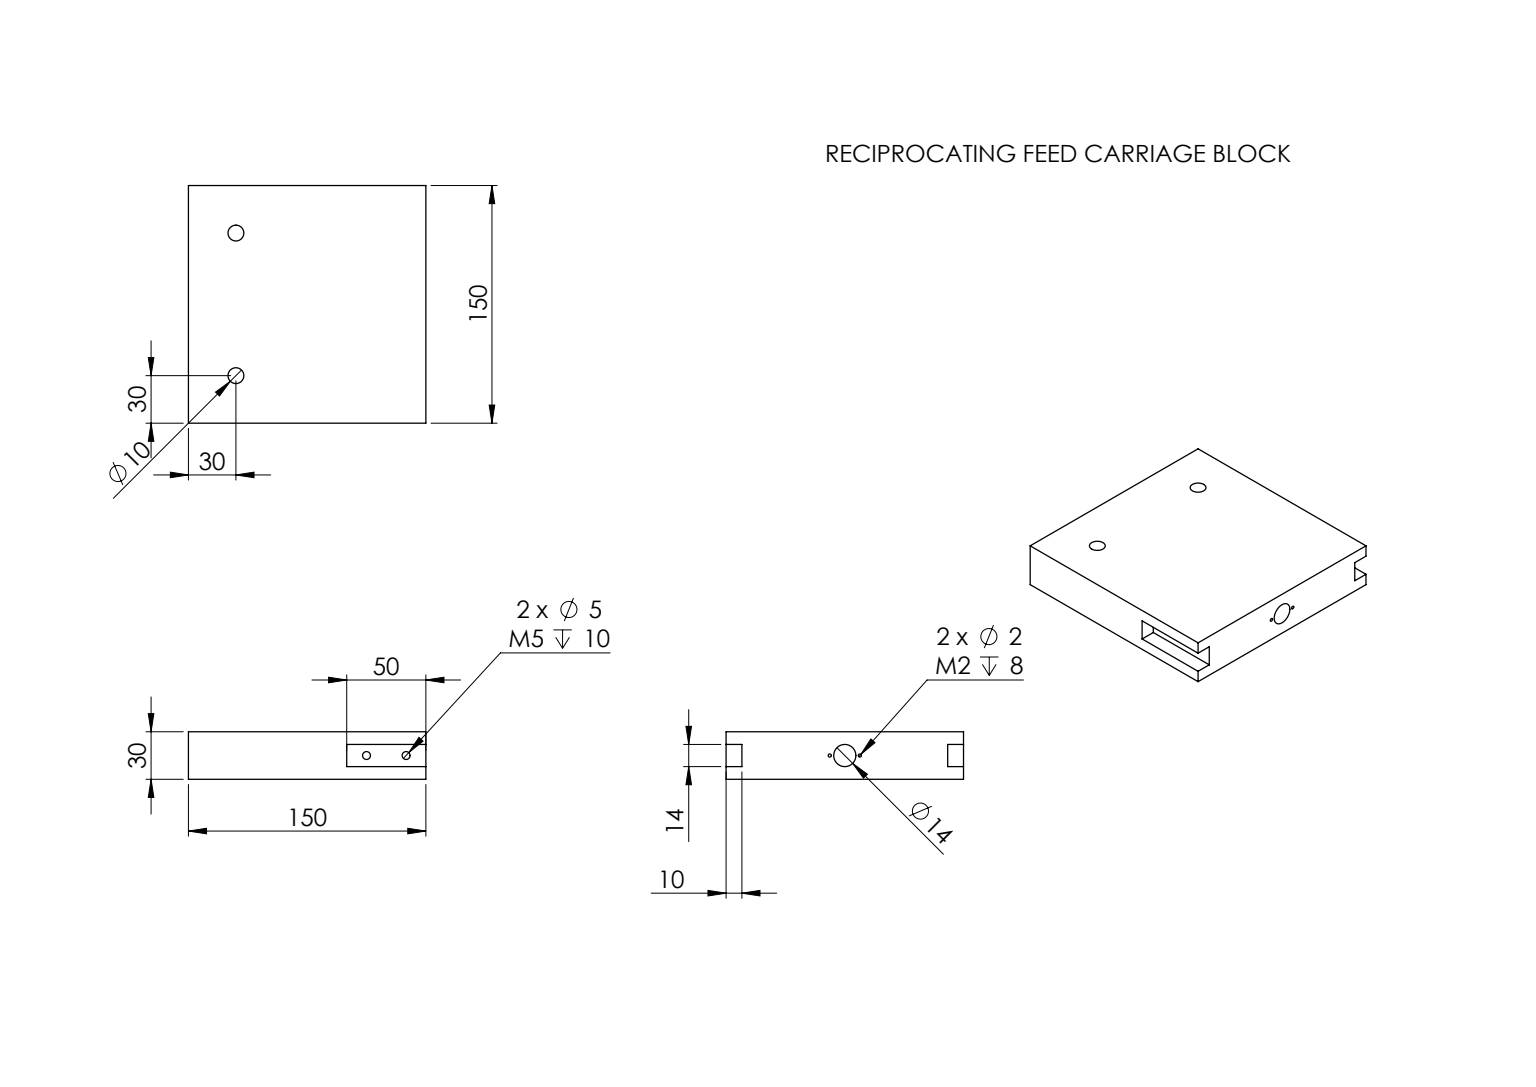
ISO-10303-21;
HEADER;
FILE_DESCRIPTION (('STEP AP214'),
    '1' );
FILE_NAME ('Reciprocating Feed Carriage Block.step',
    '2026-10-27T14:18:53',
    ( '' ),
    ( '' ),
    'SwSTEP 2.0',
    'SolidWorks 2026',
    '' );
FILE_SCHEMA (( 'AUTOMOTIVE_DESIGN' ));
ENDSEC;

DATA;
#3=LINE ( 'NONE', #3246, #2138 ) ;
#4=EDGE_LOOP ( 'NONE', ( #1502, #1673, #5385 ) ) ;
#6=FACE_BOUND ( 'NONE', #2071, .T. ) ;
#7=AXIS2_PLACEMENT_3D ( 'NONE', #5540, #5177, #924 ) ;
#19=DIRECTION ( 'NONE',  ( 0.8571673013836870192, 1.049727191973306873E-16, -0.5150380737757234151 ) ) ;
#21=VECTOR ( 'NONE', #291, 1000.000000000000000 ) ;
#22=EDGE_LOOP ( 'NONE', ( #259, #3713, #2794, #1342 ) ) ;
#23=ADVANCED_FACE ( 'NONE', ( #3966 ), #1603, .F. ) ;
#24=ORIENTED_EDGE ( 'NONE', *, *, #4586, .F. ) ;
#25=CIRCLE ( 'NONE', #2627, 2.500000000000002220 ) ;
#28=DIRECTION ( 'NONE',  ( 1.000000000000000000, -0.000000000000000000, -0.000000000000000000 ) ) ;
#30=CARTESIAN_POINT ( 'NONE',  ( 25.00000000000000711, 7.000000000000011546, 65.00000000000000000 ) ) ;
#33=CIRCLE ( 'NONE', #3411, 2.500000000000002220 ) ;
#34=VECTOR ( 'NONE', #480, 1000.000000000000000 ) ;
#39=EDGE_CURVE ( 'NONE', #3671, #1708, #102, .T. ) ;
#41=ORIENTED_EDGE ( 'NONE', *, *, #5391, .F. ) ;
#45=CARTESIAN_POINT ( 'NONE',  ( 55.00000000000000711, 0.000000000000000000, 0.000000000000000000 ) ) ;
#55=EDGE_CURVE ( 'NONE', #1875, #2958, #1837, .T. ) ;
#56=CARTESIAN_POINT ( 'NONE',  ( -45.00000000000002842, 0.000000000000000000, -49.99999999999998579 ) ) ;
#58=PRODUCT ( 'Reciprocating Feed Carriage Block', 'Reciprocating Feed Carriage Block', '', ( #3675 ) ) ;
#59=DIRECTION ( 'NONE',  ( 0.000000000000000000, 0.000000000000000000, 1.000000000000000000 ) ) ;
#61=ADVANCED_FACE ( 'NONE', ( #5096 ), #2836, .F. ) ;
#66=DIRECTION ( 'NONE',  ( 1.000000000000000000, 0.000000000000000000, 0.000000000000000000 ) ) ;
#70=ADVANCED_FACE ( 'NONE', ( #1406 ), #469, .F. ) ;
#72=EDGE_LOOP ( 'NONE', ( #5163, #1445, #4342, #1553 ) ) ;
#77=ORIENTED_EDGE ( 'NONE', *, *, #5201, .F. ) ;
#81=ORIENTED_EDGE ( 'NONE', *, *, #5316, .T. ) ;
#90=CARTESIAN_POINT ( 'NONE',  ( 75.00000000000001421, 0.000000000000000000, 0.000000000000000000 ) ) ;
#100=FACE_OUTER_BOUND ( 'NONE', #830, .T. ) ;
#102=CIRCLE ( 'NONE', #5140, 2.500000000000002220 ) ;
#115=DIRECTION ( 'NONE',  ( -0.000000000000000000, -0.000000000000000000, 1.000000000000000000 ) ) ;
#116=DIRECTION ( 'NONE',  ( 1.000000000000000000, -0.000000000000000000, -0.000000000000000000 ) ) ;
#124=DIRECTION ( 'NONE',  ( 0.000000000000000000, 0.000000000000000000, -1.000000000000000000 ) ) ;
#125=CIRCLE ( 'NONE', #3997, 7.000000000000000000 ) ;
#127=EDGE_LOOP ( 'NONE', ( #1000, #825, #2890, #4264 ) ) ;
#139=EDGE_LOOP ( 'NONE', ( #819, #2768, #3895, #5842 ) ) ;
#141=EDGE_CURVE ( 'NONE', #5390, #1345, #2004, .T. ) ;
#146=ORIENTED_EDGE ( 'NONE', *, *, #1899, .T. ) ;
#151=CARTESIAN_POINT ( 'NONE',  ( 75.00000000000001421, 1.224646799147354440E-16, -8.500000000000000000 ) ) ;
#166=ORIENTED_EDGE ( 'NONE', *, *, #2504, .F. ) ;
#168=ADVANCED_FACE ( 'NONE', ( #2861 ), #5707, .F. ) ;
#183=ORIENTED_EDGE ( 'NONE', *, *, #1823, .F. ) ;
#190=DIRECTION ( 'NONE',  ( 1.000000000000000000, 0.000000000000000000, 0.000000000000000000 ) ) ;
#197=CARTESIAN_POINT ( 'NONE',  ( 37.50000000000000711, 6.288372600415927295E-15, 65.00000000000000000 ) ) ;
#200=DIRECTION ( 'NONE',  ( -1.000000000000000000, 2.312964634635742895E-17, 0.000000000000000000 ) ) ;
#201=ADVANCED_FACE ( 'NONE', ( #5199 ), #2031, .F. ) ;
#205=AXIS2_PLACEMENT_3D ( 'NONE', #3546, #4367, #1077 ) ;
#208=ADVANCED_FACE ( 'NONE', ( #1064 ), #1706, .F. ) ;
#209=LINE ( 'NONE', #2049, #935 ) ;
#215=CYLINDRICAL_SURFACE ( 'NONE', #3221, 5.000000000000004441 ) ;
#224=EDGE_CURVE ( 'NONE', #3671, #5354, #1284, .T. ) ;
#227=( NAMED_UNIT ( * ) PLANE_ANGLE_UNIT ( ) SI_UNIT ( $, .RADIAN. ) );
#228=VECTOR ( 'NONE', #4642, 1000.000000000000000 ) ;
#237=LINE ( 'NONE', #652, #2519 ) ;
#238=DIRECTION ( 'NONE',  ( 0.000000000000000000, 1.000000000000000000, -0.000000000000000000 ) ) ;
#245=DIRECTION ( 'NONE',  ( 1.000000000000000000, -0.000000000000000000, -0.000000000000000000 ) ) ;
#246=DIRECTION ( 'NONE',  ( -0.000000000000000000, -0.000000000000000000, -1.000000000000000000 ) ) ;
#251=ORIENTED_EDGE ( 'NONE', *, *, #3575, .F. ) ;
#253=ORIENTED_EDGE ( 'NONE', *, *, #2086, .T. ) ;
#254=ADVANCED_FACE ( 'NONE', ( #5836 ), #1248, .F. ) ;
#255=LINE ( 'NONE', #2124, #1542 ) ;
#259=ORIENTED_EDGE ( 'NONE', *, *, #388, .T. ) ;
#262=DIRECTION ( 'NONE',  ( 1.000000000000000000, -0.000000000000000000, -0.000000000000000000 ) ) ;
#268=CYLINDRICAL_SURFACE ( 'NONE', #4477, 2.500000000000002220 ) ;
#273=ORIENTED_EDGE ( 'NONE', *, *, #4438, .F. ) ;
#283=VERTEX_POINT ( 'NONE', #413 ) ;
#286=ORIENTED_EDGE ( 'NONE', *, *, #1877, .F. ) ;
#290=ORIENTED_EDGE ( 'NONE', *, *, #4030, .T. ) ;
#291=DIRECTION ( 'NONE',  ( 1.000000000000000000, -3.469446951953614189E-16, -0.000000000000000000 ) ) ;
#299=FACE_OUTER_BOUND ( 'NONE', #2161, .T. ) ;
#305=VECTOR ( 'NONE', #5098, 1000.000000000000000 ) ;
#306=DIRECTION ( 'NONE',  ( 0.000000000000000000, 0.000000000000000000, 1.000000000000000000 ) ) ;
#311=ADVANCED_FACE ( 'NONE', ( #2255 ), #3623, .F. ) ;
#312=DIRECTION ( 'NONE',  ( 1.000000000000000000, 0.000000000000000000, -0.000000000000000000 ) ) ;
#315=EDGE_CURVE ( 'NONE', #2436, #2440, #3153, .T. ) ;
#316=EDGE_CURVE ( 'NONE', #4485, #2436, #3260, .T. ) ;
#326=ORIENTED_EDGE ( 'NONE', *, *, #3762, .T. ) ;
#328=DIRECTION ( 'NONE',  ( 1.000000000000000000, -0.000000000000000000, -0.000000000000000000 ) ) ;
#329=EDGE_LOOP ( 'NONE', ( #3488, #1309 ) ) ;
#344=ORIENTED_EDGE ( 'NONE', *, *, #547, .F. ) ;
#351=ORIENTED_EDGE ( 'NONE', *, *, #1899, .F. ) ;
#352=DIRECTION ( 'NONE',  ( -1.000000000000000000, 0.000000000000000000, 0.000000000000000000 ) ) ;
#353=DIRECTION ( 'NONE',  ( -0.000000000000000000, -0.000000000000000000, 1.000000000000000000 ) ) ;
#354=EDGE_LOOP ( 'NONE', ( #2724, #1394 ) ) ;
#356=CARTESIAN_POINT ( 'NONE',  ( -74.99999999999998579, 15.00000000000000000, 75.00000000000000000 ) ) ;
#357=ORIENTED_EDGE ( 'NONE', *, *, #4065, .T. ) ;
#360=VERTEX_POINT ( 'NONE', #5089 ) ;
#365=DIRECTION ( 'NONE',  ( -0.000000000000000000, -0.000000000000000000, 1.000000000000000000 ) ) ;
#368=EDGE_LOOP ( 'NONE', ( #4286, #2908, #2582, #3247 ) ) ;
#369=CARTESIAN_POINT ( 'NONE',  ( -45.00000000000002842, 15.00000000000000000, -39.99999999999997868 ) ) ;
#372=ADVANCED_FACE ( 'NONE', ( #1311 ), #889, .T. ) ;
#380=DIRECTION ( 'NONE',  ( -3.469446951953614189E-16, -1.000000000000000000, 8.673617379884041635E-17 ) ) ;
#383=LINE ( 'NONE', #2712, #21 ) ;
#386=VECTOR ( 'NONE', #1556, 1000.000000000000000 ) ;
#388=EDGE_CURVE ( 'NONE', #475, #702, #3140, .T. ) ;
#389=CARTESIAN_POINT ( 'NONE',  ( 25.00000000000000711, 7.000000000000011546, -75.00000000000000000 ) ) ;
#390=EDGE_CURVE ( 'NONE', #5094, #2958, #1969, .T. ) ;
#398=DIRECTION ( 'NONE',  ( 1.000000000000000000, -0.000000000000000000, -0.000000000000000000 ) ) ;
#399=AXIS2_PLACEMENT_3D ( 'NONE', #949, #5510, #3267 ) ;
#400=VECTOR ( 'NONE', #539, 1000.000000000000000 ) ;
#402=FACE_BOUND ( 'NONE', #4375, .T. ) ;
#404=LINE ( 'NONE', #5952, #3410 ) ;
#413=CARTESIAN_POINT ( 'NONE',  ( 62.50000000000001421, -1.951563910473909559E-15, -53.49784845693390167 ) ) ;
#416=AXIS2_PLACEMENT_3D ( 'NONE', #5969, #3664, #3218 ) ;
#428=ORIENTED_EDGE ( 'NONE', *, *, #4995, .T. ) ;
#436=CARTESIAN_POINT ( 'NONE',  ( 62.50000000000001421, -1.951563910473909559E-15, -65.00000000000000000 ) ) ;
#444=ORIENTED_EDGE ( 'NONE', *, *, #5201, .T. ) ;
#445=DIRECTION ( 'NONE',  ( -0.000000000000000000, -0.000000000000000000, 1.000000000000000000 ) ) ;
#447=ORIENTED_EDGE ( 'NONE', *, *, #1010, .T. ) ;
#452=DIRECTION ( 'NONE',  ( -0.000000000000000000, -0.000000000000000000, -1.000000000000000000 ) ) ;
#453=ORIENTED_EDGE ( 'NONE', *, *, #824, .F. ) ;
#459=ADVANCED_FACE ( 'NONE', ( #1056 ), #3071, .F. ) ;
#469=CYLINDRICAL_SURFACE ( 'NONE', #580, 5.000000000000004441 ) ;
#475=VERTEX_POINT ( 'NONE', #614 ) ;
#476=CIRCLE ( 'NONE', #7, 5.000000000000004441 ) ;
#480=DIRECTION ( 'NONE',  ( 1.000000000000000000, -3.469446951953614189E-16, 0.000000000000000000 ) ) ;
#482=ORIENTED_EDGE ( 'NONE', *, *, #2535, .F. ) ;
#484=CONICAL_SURFACE ( 'NONE', #5051, 2.500000000000002220, 1.029744260000002631 ) ;
#501=DIRECTION ( 'NONE',  ( 1.000000000000000000, -0.000000000000000000, -0.000000000000000000 ) ) ;
#503=VECTOR ( 'NONE', #5031, 1000.000000000000000 ) ;
#507=FACE_OUTER_BOUND ( 'NONE', #3343, .T. ) ;
#512=CARTESIAN_POINT ( 'NONE',  ( 75.00000000000001421, 6.999999999999993783, 65.00000000000000000 ) ) ;
#518=AXIS2_PLACEMENT_3D ( 'NONE', #4463, #3550, #3968 ) ;
#520=CYLINDRICAL_SURFACE ( 'NONE', #602, 7.000000000000000000 ) ;
#524=ORIENTED_EDGE ( 'NONE', *, *, #4694, .F. ) ;
#525=VERTEX_POINT ( 'NONE', #3821 ) ;
#528=EDGE_CURVE ( 'NONE', #4999, #2390, #5702, .T. ) ;
#535=EDGE_LOOP ( 'NONE', ( #1085, #4060 ) ) ;
#539=DIRECTION ( 'NONE',  ( 0.8571673013836870192, 1.049727191973306873E-16, -0.5150380737757234151 ) ) ;
#543=EDGE_LOOP ( 'NONE', ( #1731, #977, #5859, #3323 ) ) ;
#547=EDGE_CURVE ( 'NONE', #3406, #1861, #2828, .T. ) ;
#550=DIRECTION ( 'NONE',  ( -0.000000000000000000, -0.000000000000000000, 1.000000000000000000 ) ) ;
#554=VERTEX_POINT ( 'NONE', #5768 ) ;
#555=APPLICATION_CONTEXT ( 'automotive_design' ) ;
#558=DIRECTION ( 'NONE',  ( 0.5150380737757185301, 0.000000000000000000, -0.8571673013836900168 ) ) ;
#568=DIRECTION ( 'NONE',  ( 0.000000000000000000, -1.734723475976808080E-16, 1.000000000000000000 ) ) ;
#572=CARTESIAN_POINT ( 'NONE',  ( 62.50000000000001421, -1.951563910473909559E-15, 65.00000000000000000 ) ) ;
#574=CIRCLE ( 'NONE', #1347, 2.500000000000002220 ) ;
#580=AXIS2_PLACEMENT_3D ( 'NONE', #923, #899, #1346 ) ;
#582=CIRCLE ( 'NONE', #3972, 5.000000000000004441 ) ;
#589=ORIENTED_EDGE ( 'NONE', *, *, #2162, .T. ) ;
#592=LINE ( 'NONE', #3245, #305 ) ;
#600=CARTESIAN_POINT ( 'NONE',  ( 40.00000000000000711, 6.594534300202765954E-15, -55.00000000000000000 ) ) ;
#602=AXIS2_PLACEMENT_3D ( 'NONE', #45, #5111, #4256 ) ;
#603=DIRECTION ( 'NONE',  ( 0.8571673013836870192, 0.000000000000000000, 0.5150380737757234151 ) ) ;
#611=EDGE_CURVE ( 'NONE', #5793, #5838, #2551, .T. ) ;
#614=CARTESIAN_POINT ( 'NONE',  ( -74.99999999999998579, 15.00000000000000000, -75.00000000000000000 ) ) ;
#632=FACE_OUTER_BOUND ( 'NONE', #5560, .T. ) ;
#636=LINE ( 'NONE', #1087, #4113 ) ;
#639=SURFACE_STYLE_USAGE ( .BOTH. , #1582 ) ;
#640=EDGE_CURVE ( 'NONE', #3205, #5222, #255, .T. ) ;
#646=ADVANCED_FACE ( 'NONE', ( #1584 ), #3437, .T. ) ;
#648=ORIENTED_EDGE ( 'NONE', *, *, #3065, .F. ) ;
#650=ORIENTED_EDGE ( 'NONE', *, *, #39, .T. ) ;
#652=CARTESIAN_POINT ( 'NONE',  ( 60.00000000000001421, -1.951563910473909559E-15, -65.00000000000000000 ) ) ;
#667=DIRECTION ( 'NONE',  ( 1.000000000000000000, 0.000000000000000000, 0.000000000000000000 ) ) ;
#678=DIRECTION ( 'NONE',  ( 0.000000000000000000, 0.000000000000000000, -1.000000000000000000 ) ) ;
#680=FACE_OUTER_BOUND ( 'NONE', #139, .T. ) ;
#683=CARTESIAN_POINT ( 'NONE',  ( 55.00000000000000711, 0.000000000000000000, 0.000000000000000000 ) ) ;
#684=AXIS2_PLACEMENT_3D ( 'NONE', #5967, #4087, #2630 ) ;
#688=CIRCLE ( 'NONE', #1363, 2.500000000000002220 ) ;
#694=EDGE_CURVE ( 'NONE', #695, #4416, #2094, .T. ) ;
#695=VERTEX_POINT ( 'NONE', #1702 ) ;
#697=AXIS2_PLACEMENT_3D ( 'NONE', #1015, #2868, #3805 ) ;
#702=VERTEX_POINT ( 'NONE', #792 ) ;
#705=VECTOR ( 'NONE', #452, 1000.000000000000000 ) ;
#723=CARTESIAN_POINT ( 'NONE',  ( 37.50000000000000711, 6.288372600415927295E-15, -65.00000000000000000 ) ) ;
#726=VERTEX_POINT ( 'NONE', #5022 ) ;
#727=EDGE_CURVE ( 'NONE', #525, #782, #3196, .T. ) ;
#728=ORIENTED_EDGE ( 'NONE', *, *, #2465, .F. ) ;
#730=VECTOR ( 'NONE', #4229, 1000.000000000000000 ) ;
#732=CARTESIAN_POINT ( 'NONE',  ( 75.00000000000001421, -7.000000000000006217, 65.00000000000000000 ) ) ;
#734=DIRECTION ( 'NONE',  ( 0.5150380737757185301, 0.000000000000000000, -0.8571673013836900168 ) ) ;
#735=EDGE_LOOP ( 'NONE', ( #5844, #4817, #4105, #4046 ) ) ;
#736=VERTEX_POINT ( 'NONE', #4158 ) ;
#740=PLANE ( 'NONE',  #879 ) ;
#743=CARTESIAN_POINT ( 'NONE',  ( 75.00000000000001421, 0.000000000000000000, -9.500000000000000000 ) ) ;
#750=CARTESIAN_POINT ( 'NONE',  ( 37.50000000000000711, 6.288372600415927295E-15, -53.49784845693390167 ) ) ;
#753=EDGE_CURVE ( 'NONE', #5930, #5402, #4102, .T. ) ;
#759=CARTESIAN_POINT ( 'NONE',  ( -45.00000000000001421, 15.00000000000000000, 50.00000000000000000 ) ) ;
#774=AXIS2_PLACEMENT_3D ( 'NONE', #3204, #5115, #943 ) ;
#782=VERTEX_POINT ( 'NONE', #4645 ) ;
#788=DIRECTION ( 'NONE',  ( 0.000000000000000000, -0.000000000000000000, 1.000000000000000000 ) ) ;
#792=CARTESIAN_POINT ( 'NONE',  ( -74.99999999999998579, -15.00000000000000000, -75.00000000000000000 ) ) ;
#794=CARTESIAN_POINT ( 'NONE',  ( 25.00000000000000711, -6.999999999999989342, -75.00000000000000000 ) ) ;
#801=LINE ( 'NONE', #1707, #2409 ) ;
#804=CARTESIAN_POINT ( 'NONE',  ( -74.99999999999998579, -15.00000000000000000, 75.00000000000000000 ) ) ;
#807=ORIENTED_EDGE ( 'NONE', *, *, #4472, .F. ) ;
#815=FACE_OUTER_BOUND ( 'NONE', #1902, .T. ) ;
#819=ORIENTED_EDGE ( 'NONE', *, *, #5570, .T. ) ;
#824=EDGE_CURVE ( 'NONE', #5481, #3560, #1471, .T. ) ;
#825=ORIENTED_EDGE ( 'NONE', *, *, #2684, .T. ) ;
#826=EDGE_CURVE ( 'NONE', #3782, #1794, #404, .T. ) ;
#830=EDGE_LOOP ( 'NONE', ( #5101, #4107, #648, #1776 ) ) ;
#831=ADVANCED_FACE ( 'NONE', ( #1816 ), #2821, .F. ) ;
#833=CYLINDRICAL_SURFACE ( 'NONE', #3407, 5.000000000000004441 ) ;
#835=DIRECTION ( 'NONE',  ( -1.000000000000000000, 0.000000000000000000, 0.000000000000000000 ) ) ;
#847=DIRECTION ( 'NONE',  ( 0.000000000000000000, -1.000000000000000000, 0.000000000000000000 ) ) ;
#851=LINE ( 'NONE', #794, #3395 ) ;
#855=FACE_OUTER_BOUND ( 'NONE', #329, .T. ) ;
#856=EDGE_LOOP ( 'NONE', ( #5146, #4252 ) ) ;
#861=CARTESIAN_POINT ( 'NONE',  ( 40.00000000000000711, 6.288372600415927295E-15, 65.00000000000000000 ) ) ;
#874=AXIS2_PLACEMENT_3D ( 'NONE', #5482, #501, #5564 ) ;
#876=EDGE_CURVE ( 'NONE', #1861, #2678, #2267, .T. ) ;
#879=AXIS2_PLACEMENT_3D ( 'NONE', #3952, #1560, #200 ) ;
#889=PLANE ( 'NONE',  #5001 ) ;
#891=EDGE_LOOP ( 'NONE', ( #1245, #4583, #2532, #2172 ) ) ;
#895=DIRECTION ( 'NONE',  ( 1.000000000000000000, -0.000000000000000000, -0.000000000000000000 ) ) ;
#898=ORIENTED_EDGE ( 'NONE', *, *, #5242, .F. ) ;
#899=DIRECTION ( 'NONE',  ( 0.000000000000000000, -1.000000000000000000, 0.000000000000000000 ) ) ;
#903=CARTESIAN_POINT ( 'NONE',  ( 75.00000000000001421, 6.999999999999993783, 65.00000000000000000 ) ) ;
#905=ORIENTED_EDGE ( 'NONE', *, *, #3907, .F. ) ;
#910=EDGE_CURVE ( 'NONE', #5326, #2440, #2911, .T. ) ;
#914=CONICAL_SURFACE ( 'NONE', #4127, 0.9999999999999991118, 1.029744260000008405 ) ;
#919=CARTESIAN_POINT ( 'NONE',  ( 62.50000000000001421, -1.951563910473909559E-15, 65.00000000000000000 ) ) ;
#921=EDGE_LOOP ( 'NONE', ( #4487, #2367, #4251 ) ) ;
#923=CARTESIAN_POINT ( 'NONE',  ( -45.00000000000001421, 15.00000000000000000, 45.00000000000000000 ) ) ;
#924=DIRECTION ( 'NONE',  ( 0.000000000000000000, 0.000000000000000000, -1.000000000000000000 ) ) ;
#929=EDGE_LOOP ( 'NONE', ( #5175, #3265, #2543, #4407 ) ) ;
#935=VECTOR ( 'NONE', #5236, 1000.000000000000000 ) ;
#941=DIRECTION ( 'NONE',  ( 0.000000000000000000, 0.000000000000000000, -1.000000000000000000 ) ) ;
#943=DIRECTION ( 'NONE',  ( 1.000000000000000000, 0.000000000000000000, 0.000000000000000000 ) ) ;
#949=CARTESIAN_POINT ( 'NONE',  ( -45.00000000000002842, 0.000000000000000000, -44.99999999999998579 ) ) ;
#958=DIRECTION ( 'NONE',  ( 1.000000000000000000, 0.000000000000000000, 0.000000000000000000 ) ) ;
#969=VECTOR ( 'NONE', #5788, 1000.000000000000000 ) ;
#971=EDGE_CURVE ( 'NONE', #3782, #4485, #636, .T. ) ;
#974=DIRECTION ( 'NONE',  ( 0.000000000000000000, 0.000000000000000000, -1.000000000000000000 ) ) ;
#977=ORIENTED_EDGE ( 'NONE', *, *, #4586, .T. ) ;
#984=STYLED_ITEM('',(#5999),#4254);
#998=ORIENTED_EDGE ( 'NONE', *, *, #2662, .F. ) ;
#1000=ORIENTED_EDGE ( 'NONE', *, *, #2050, .F. ) ;
#1002=DIRECTION ( 'NONE',  ( 1.000000000000000000, 0.000000000000000000, 0.000000000000000000 ) ) ;
#1004=FACE_OUTER_BOUND ( 'NONE', #921, .T. ) ;
#1008=EDGE_CURVE ( 'NONE', #5390, #475, #3912, .T. ) ;
#1009=EDGE_LOOP ( 'NONE', ( #3834, #3467, #2612, #4538 ) ) ;
#1010=EDGE_CURVE ( 'NONE', #5437, #4485, #1606, .T. ) ;
#1015=CARTESIAN_POINT ( 'NONE',  ( 55.00000000000000711, 0.000000000000000000, 0.000000000000000000 ) ) ;
#1022=EDGE_CURVE ( 'NONE', #3819, #5507, #5764, .T. ) ;
#1023=CARTESIAN_POINT ( 'NONE',  ( 75.00000000000001421, 6.999999999999993783, -65.00000000000000000 ) ) ;
#1024=ADVANCED_FACE ( 'NONE', ( #5313, #2547, #1115 ), #5854, .F. ) ;
#1029=CARTESIAN_POINT ( 'NONE',  ( 67.00000000000000000, 0.000000000000000000, -9.500000000000000000 ) ) ;
#1032=CARTESIAN_POINT ( 'NONE',  ( 60.00000000000001421, -1.645402210687070900E-15, 55.00000000000000000 ) ) ;
#1035=CARTESIAN_POINT ( 'NONE',  ( 62.50000000000001421, -1.951563910473909559E-15, -55.00000000000000000 ) ) ;
#1041=VERTEX_POINT ( 'NONE', #3522 ) ;
#1044=LINE ( 'NONE', #600, #400 ) ;
#1046=CARTESIAN_POINT ( 'NONE',  ( 25.00000000000000711, -6.999999999999988454, -65.00000000000000000 ) ) ;
#1047=EDGE_LOOP ( 'NONE', ( #2451, #5773, #650 ) ) ;
#1054=AXIS2_PLACEMENT_3D ( 'NONE', #1824, #1337, #2748 ) ;
#1056=FACE_OUTER_BOUND ( 'NONE', #1413, .T. ) ;
#1064=FACE_OUTER_BOUND ( 'NONE', #5144, .T. ) ;
#1068=FACE_BOUND ( 'NONE', #4272, .T. ) ;
#1069=DIRECTION ( 'NONE',  ( -0.000000000000000000, -0.000000000000000000, -1.000000000000000000 ) ) ;
#1077=DIRECTION ( 'NONE',  ( -1.000000000000000000, 0.000000000000000000, 0.000000000000000000 ) ) ;
#1082=EDGE_CURVE ( 'NONE', #1794, #2436, #4374, .T. ) ;
#1084=ADVANCED_FACE ( 'NONE', ( #4924 ), #4437, .F. ) ;
#1085=ORIENTED_EDGE ( 'NONE', *, *, #4472, .T. ) ;
#1087=CARTESIAN_POINT ( 'NONE',  ( 25.00000000000000711, 7.000000000000011546, -65.00000000000000000 ) ) ;
#1088=MECHANICAL_DESIGN_GEOMETRIC_PRESENTATION_REPRESENTATION('',(#3609),#4496);
#1091=DIRECTION ( 'NONE',  ( 1.000000000000000000, -0.000000000000000000, -0.000000000000000000 ) ) ;
#1111=LINE ( 'NONE', #4823, #969 ) ;
#1112=ORIENTED_EDGE ( 'NONE', *, *, #5912, .T. ) ;
#1115=FACE_OUTER_BOUND ( 'NONE', #2487, .T. ) ;
#1121=DIRECTION ( 'NONE',  ( -0.000000000000000000, 0.000000000000000000, -1.000000000000000000 ) ) ;
#1128=ORIENTED_EDGE ( 'NONE', *, *, #2566, .T. ) ;
#1129=FACE_OUTER_BOUND ( 'NONE', #127, .T. ) ;
#1136=CARTESIAN_POINT ( 'NONE',  ( 37.50000000000000711, 6.288372600415927295E-15, 53.49784845693390167 ) ) ;
#1137=DIRECTION ( 'NONE',  ( -0.000000000000000000, 8.673617379884040402E-17, -1.000000000000000000 ) ) ;
#1141=DIRECTION ( 'NONE',  ( -1.000000000000000000, 0.000000000000000000, 0.000000000000000000 ) ) ;
#1157=DIRECTION ( 'NONE',  ( 1.000000000000000000, 0.000000000000000000, 0.000000000000000000 ) ) ;
#1158=DIRECTION ( 'NONE',  ( 0.000000000000000000, -1.000000000000000000, 0.000000000000000000 ) ) ;
#1160=LINE ( 'NONE', #5752, #5538 ) ;
#1162=ORIENTED_EDGE ( 'NONE', *, *, #2458, .T. ) ;
#1167=DIRECTION ( 'NONE',  ( -1.000000000000000000, 0.000000000000000000, 0.000000000000000000 ) ) ;
#1169=DIRECTION ( 'NONE',  ( 1.000000000000000000, -0.000000000000000000, -0.000000000000000000 ) ) ;
#1175=VERTEX_POINT ( 'NONE', #369 ) ;
#1181=CONICAL_SURFACE ( 'NONE', #4874, 0.9999999999999991118, 1.029744260000008405 ) ;
#1182=( NAMED_UNIT ( * ) SI_UNIT ( $, .STERADIAN. ) SOLID_ANGLE_UNIT ( ) );
#1186=ORIENTED_EDGE ( 'NONE', *, *, #4972, .F. ) ;
#1192=ORIENTED_EDGE ( 'NONE', *, *, #4065, .F. ) ;
#1194=DIRECTION ( 'NONE',  ( -1.000000000000000000, -0.000000000000000000, -0.000000000000000000 ) ) ;
#1196=ORIENTED_EDGE ( 'NONE', *, *, #4877, .T. ) ;
#1197=LINE ( 'NONE', #5931, #2731 ) ;
#1199=ORIENTED_EDGE ( 'NONE', *, *, #2684, .F. ) ;
#1203=DIRECTION ( 'NONE',  ( 0.000000000000000000, 0.000000000000000000, -1.000000000000000000 ) ) ;
#1204=DIRECTION ( 'NONE',  ( 0.000000000000000000, 1.000000000000000000, -0.000000000000000000 ) ) ;
#1205=DIRECTION ( 'NONE',  ( 0.000000000000000000, 1.000000000000000000, 0.000000000000000000 ) ) ;
#1209=DIRECTION ( 'NONE',  ( 1.000000000000000000, -3.469446951953614189E-16, 0.000000000000000000 ) ) ;
#1210=ADVANCED_FACE ( 'NONE', ( #5460 ), #914, .F. ) ;
#1211=ORIENTED_EDGE ( 'NONE', *, *, #2167, .F. ) ;
#1212=( LENGTH_UNIT ( ) NAMED_UNIT ( * ) SI_UNIT ( .MILLI., .METRE. ) );
#1218=CIRCLE ( 'NONE', #2870, 7.000000000000000000 ) ;
#1221=AXIS2_PLACEMENT_3D ( 'NONE', #2854, #550, #190 ) ;
#1224=ORIENTED_EDGE ( 'NONE', *, *, #826, .F. ) ;
#1225=CARTESIAN_POINT ( 'NONE',  ( -74.99999999999998579, 15.00000000000000000, -75.00000000000000000 ) ) ;
#1231=DIRECTION ( 'NONE',  ( 0.000000000000000000, -1.734723475976808080E-16, 1.000000000000000000 ) ) ;
#1232=ADVANCED_BREP_SHAPE_REPRESENTATION ( '', ( #4254, #5080 ), #2935 ) ;
#1235=DIRECTION ( 'NONE',  ( 0.000000000000000000, 0.000000000000000000, 1.000000000000000000 ) ) ;
#1240=EDGE_LOOP ( 'NONE', ( #1618, #286, #24, #1162 ) ) ;
#1241=DIRECTION ( 'NONE',  ( 0.000000000000000000, 1.000000000000000000, 0.000000000000000000 ) ) ;
#1245=ORIENTED_EDGE ( 'NONE', *, *, #316, .F. ) ;
#1246=CIRCLE ( 'NONE', #4646, 2.500000000000002220 ) ;
#1248=CYLINDRICAL_SURFACE ( 'NONE', #2633, 2.500000000000002220 ) ;
#1254=ORIENTED_EDGE ( 'NONE', *, *, #2364, .F. ) ;
#1261=FACE_OUTER_BOUND ( 'NONE', #1992, .T. ) ;
#1268=FACE_BOUND ( 'NONE', #354, .T. ) ;
#1269=ORIENTED_EDGE ( 'NONE', *, *, #4856, .T. ) ;
#1270=ADVANCED_FACE ( 'NONE', ( #5518 ), #4128, .F. ) ;
#1275=ADVANCED_FACE ( 'NONE', ( #1268, #6, #1844 ), #3161, .F. ) ;
#1277=DIRECTION ( 'NONE',  ( 1.000000000000000000, -0.000000000000000000, -0.000000000000000000 ) ) ;
#1280=CONICAL_SURFACE ( 'NONE', #2146, 0.9999999999999991118, 1.029744260000008405 ) ;
#1281=DIRECTION ( 'NONE',  ( -0.000000000000000000, -1.000000000000000000, 0.000000000000000000 ) ) ;
#1282=ORIENTED_EDGE ( 'NONE', *, *, #2699, .F. ) ;
#1284=LINE ( 'NONE', #4387, #1450 ) ;
#1291=ORIENTED_EDGE ( 'NONE', *, *, #2604, .F. ) ;
#1296=DIRECTION ( 'NONE',  ( -0.000000000000000000, -0.000000000000000000, 1.000000000000000000 ) ) ;
#1309=ORIENTED_EDGE ( 'NONE', *, *, #3862, .T. ) ;
#1311=FACE_OUTER_BOUND ( 'NONE', #1979, .T. ) ;
#1323=LINE ( 'NONE', #3088, #3995 ) ;
#1333=ORIENTED_EDGE ( 'NONE', *, *, #547, .T. ) ;
#1337=DIRECTION ( 'NONE',  ( -0.000000000000000000, -0.000000000000000000, 1.000000000000000000 ) ) ;
#1340=CARTESIAN_POINT ( 'NONE',  ( 67.00000000000000000, 0.000000000000000000, 9.500000000000000000 ) ) ;
#1342=ORIENTED_EDGE ( 'NONE', *, *, #1008, .T. ) ;
#1343=DIRECTION ( 'NONE',  ( -0.8571673013836870192, 0.000000000000000000, -0.5150380737757234151 ) ) ;
#1344=EDGE_CURVE ( 'NONE', #5222, #2390, #1218, .T. ) ;
#1345=VERTEX_POINT ( 'NONE', #3727 ) ;
#1346=DIRECTION ( 'NONE',  ( 0.000000000000000000, 0.000000000000000000, -1.000000000000000000 ) ) ;
#1347=AXIS2_PLACEMENT_3D ( 'NONE', #2165, #353, #4567 ) ;
#1348=EDGE_CURVE ( 'NONE', #5607, #2228, #2969, .T. ) ;
#1363=AXIS2_PLACEMENT_3D ( 'NONE', #4854, #3962, #2998 ) ;
#1364=AXIS2_PLACEMENT_3D ( 'NONE', #919, #445, #1375 ) ;
#1369=CARTESIAN_POINT ( 'NONE',  ( -74.99999999999998579, -15.00000000000000000, -75.00000000000000000 ) ) ;
#1375=DIRECTION ( 'NONE',  ( 1.000000000000000000, 0.000000000000000000, 0.000000000000000000 ) ) ;
#1377=EDGE_LOOP ( 'NONE', ( #2986, #2188, #5509, #3049 ) ) ;
#1389=EDGE_CURVE ( 'NONE', #525, #4209, #1870, .T. ) ;
#1394=ORIENTED_EDGE ( 'NONE', *, *, #5599, .F. ) ;
#1397=ORIENTED_EDGE ( 'NONE', *, *, #2208, .T. ) ;
#1398=DIRECTION ( 'NONE',  ( 0.000000000000000000, 0.000000000000000000, -1.000000000000000000 ) ) ;
#1400=DIRECTION ( 'NONE',  ( 0.000000000000000000, 0.000000000000000000, -1.000000000000000000 ) ) ;
#1406=FACE_OUTER_BOUND ( 'NONE', #2930, .T. ) ;
#1413=EDGE_LOOP ( 'NONE', ( #5214, #4830, #4305 ) ) ;
#1415=CARTESIAN_POINT ( 'NONE',  ( 60.00000000000001421, -1.645402210687070900E-15, 55.00000000000000000 ) ) ;
#1423=ORIENTED_EDGE ( 'NONE', *, *, #5137, .F. ) ;
#1426=VERTEX_POINT ( 'NONE', #5184 ) ;
#1440=CIRCLE ( 'NONE', #5606, 2.500000000000002220 ) ;
#1445=ORIENTED_EDGE ( 'NONE', *, *, #640, .T. ) ;
#1450=VECTOR ( 'NONE', #3143, 1000.000000000000000 ) ;
#1452=AXIS2_PLACEMENT_3D ( 'NONE', #2467, #3052, #4841 ) ;
#1457=AXIS2_PLACEMENT_3D ( 'NONE', #3063, #4921, #5397 ) ;
#1459=CARTESIAN_POINT ( 'NONE',  ( 35.00000000000000000, 6.288372600415927295E-15, -55.00000000000000000 ) ) ;
#1463=ORIENTED_EDGE ( 'NONE', *, *, #5150, .F. ) ;
#1464=CIRCLE ( 'NONE', #416, 2.500000000000002220 ) ;
#1466=DIRECTION ( 'NONE',  ( 1.000000000000000000, -3.469446951953614189E-16, -0.000000000000000000 ) ) ;
#1471=CIRCLE ( 'NONE', #4873, 2.500000000000002220 ) ;
#1473=AXIS2_PLACEMENT_3D ( 'NONE', #5671, #1547, #5639 ) ;
#1486=ORIENTED_EDGE ( 'NONE', *, *, #5242, .T. ) ;
#1497=ORIENTED_EDGE ( 'NONE', *, *, #5150, .T. ) ;
#1498=CARTESIAN_POINT ( 'NONE',  ( 55.00000000000000711, 8.572527594031473190E-16, 7.000000000000000000 ) ) ;
#1501=CARTESIAN_POINT ( 'NONE',  ( -45.00000000000002842, 0.000000000000000000, -44.99999999999998579 ) ) ;
#1502=ORIENTED_EDGE ( 'NONE', *, *, #4106, .F. ) ;
#1503=EDGE_CURVE ( 'NONE', #5450, #5793, #209, .T. ) ;
#1510=ORIENTED_EDGE ( 'NONE', *, *, #2364, .T. ) ;
#1512=DIRECTION ( 'NONE',  ( 0.000000000000000000, 0.000000000000000000, 1.000000000000000000 ) ) ;
#1522=DIRECTION ( 'NONE',  ( 1.000000000000000000, 0.000000000000000000, 0.000000000000000000 ) ) ;
#1527=CARTESIAN_POINT ( 'NONE',  ( 35.00000000000000000, 6.594534300202765954E-15, 65.00000000000000000 ) ) ;
#1534=DIRECTION ( 'NONE',  ( 1.000000000000000000, -3.469446951953614189E-16, 0.000000000000000000 ) ) ;
#1536=CARTESIAN_POINT ( 'NONE',  ( -45.00000000000002842, 15.00000000000000000, -44.99999999999998579 ) ) ;
#1537=ORIENTED_EDGE ( 'NONE', *, *, #1872, .F. ) ;
#1538=DIRECTION ( 'NONE',  ( -0.000000000000000000, -0.000000000000000000, 1.000000000000000000 ) ) ;
#1540=UNCERTAINTY_MEASURE_WITH_UNIT (LENGTH_MEASURE( 1.000000000000000082E-05 ), #2550, 'distance_accuracy_value', 'NONE');
#1542=VECTOR ( 'NONE', #1642, 1000.000000000000000 ) ;
#1546=VECTOR ( 'NONE', #3946, 1000.000000000000114 ) ;
#1547=DIRECTION ( 'NONE',  ( 3.469446951953614189E-16, 1.000000000000000000, 1.734723475976808327E-16 ) ) ;
#1548=CARTESIAN_POINT ( 'NONE',  ( 55.00000000000000711, 0.000000000000000000, -7.000000000000000000 ) ) ;
#1549=AXIS2_PLACEMENT_3D ( 'NONE', #1035, #2891, #4297 ) ;
#1553=ORIENTED_EDGE ( 'NONE', *, *, #528, .F. ) ;
#1555=DIRECTION ( 'NONE',  ( -3.469446951953614189E-16, -1.000000000000000000, -8.673617379884041635E-17 ) ) ;
#1556=DIRECTION ( 'NONE',  ( 0.000000000000000000, 1.000000000000000000, 0.000000000000000000 ) ) ;
#1560=DIRECTION ( 'NONE',  ( 2.312964634635742895E-17, 1.000000000000000000, -0.000000000000000000 ) ) ;
#1570=DIRECTION ( 'NONE',  ( -1.000000000000000000, 0.000000000000000000, 0.000000000000000000 ) ) ;
#1575=( GEOMETRIC_REPRESENTATION_CONTEXT ( 3 ) GLOBAL_UNCERTAINTY_ASSIGNED_CONTEXT ( ( #4283 ) ) GLOBAL_UNIT_ASSIGNED_CONTEXT ( ( #1212, #2577, #2121 ) ) REPRESENTATION_CONTEXT ( 'NONE', 'WORKASPACE' ) );
#1576=VERTEX_POINT ( 'NONE', #4364 ) ;
#1579=AXIS2_PLACEMENT_3D ( 'NONE', #3650, #941, #5113 ) ;
#1581=ORIENTED_EDGE ( 'NONE', *, *, #3788, .T. ) ;
#1582=SURFACE_SIDE_STYLE ('',( #3883 ) ) ;
#1584=FACE_OUTER_BOUND ( 'NONE', #543, .T. ) ;
#1589=ORIENTED_EDGE ( 'NONE', *, *, #5731, .T. ) ;
#1590=CARTESIAN_POINT ( 'NONE',  ( -74.99999999999998579, -15.00000000000000000, 75.00000000000000000 ) ) ;
#1591=CARTESIAN_POINT ( 'NONE',  ( 75.00000000000001421, -15.00000000000000355, -75.00000000000000000 ) ) ;
#1600=LINE ( 'NONE', #2905, #2927 ) ;
#1603=CYLINDRICAL_SURFACE ( 'NONE', #5433, 0.9999999999999991118 ) ;
#1606=LINE ( 'NONE', #5820, #5473 ) ;
#1616=DIRECTION ( 'NONE',  ( 1.000000000000000000, 0.000000000000000000, 0.000000000000000000 ) ) ;
#1618=ORIENTED_EDGE ( 'NONE', *, *, #694, .T. ) ;
#1623=CARTESIAN_POINT ( 'NONE',  ( 62.50000000000001421, -1.951563910473909559E-15, 55.00000000000000000 ) ) ;
#1626=CARTESIAN_POINT ( 'NONE',  ( 66.39913938277356920, 0.000000000000000000, -9.500000000000000000 ) ) ;
#1642=DIRECTION ( 'NONE',  ( 1.000000000000000000, -0.000000000000000000, -0.000000000000000000 ) ) ;
#1648=ORIENTED_EDGE ( 'NONE', *, *, #1008, .F. ) ;
#1664=DIRECTION ( 'NONE',  ( 1.000000000000000000, 0.000000000000000000, 0.000000000000000000 ) ) ;
#1672=VECTOR ( 'NONE', #1137, 1000.000000000000000 ) ;
#1673=ORIENTED_EDGE ( 'NONE', *, *, #5391, .T. ) ;
#1685=LINE ( 'NONE', #804, #3310 ) ;
#1699=VERTEX_POINT ( 'NONE', #5897 ) ;
#1702=CARTESIAN_POINT ( 'NONE',  ( 75.00000000000001421, -7.000000000000007105, 75.00000000000000000 ) ) ;
#1706=CYLINDRICAL_SURFACE ( 'NONE', #5712, 5.000000000000004441 ) ;
#1707=CARTESIAN_POINT ( 'NONE',  ( 35.00000000000000000, 6.594534300202765954E-15, 55.00000000000000000 ) ) ;
#1708=VERTEX_POINT ( 'NONE', #5394 ) ;
#1719=CARTESIAN_POINT ( 'NONE',  ( 25.00000000000000711, 7.000000000000011546, 65.00000000000000000 ) ) ;
#1720=CARTESIAN_POINT ( 'NONE',  ( 62.50000000000001421, -1.951563910473909559E-15, 65.00000000000000000 ) ) ;
#1721=DIRECTION ( 'NONE',  ( 0.000000000000000000, 1.000000000000000000, -0.000000000000000000 ) ) ;
#1730=LINE ( 'NONE', #5352, #5232 ) ;
#1731=ORIENTED_EDGE ( 'NONE', *, *, #2906, .T. ) ;
#1732=AXIS2_PLACEMENT_3D ( 'NONE', #2985, #4838, #678 ) ;
#1737=DIRECTION ( 'NONE',  ( 0.000000000000000000, 0.000000000000000000, -1.000000000000000000 ) ) ;
#1743=CARTESIAN_POINT ( 'NONE',  ( 75.00000000000001421, 0.000000000000000000, 9.500000000000000000 ) ) ;
#1749=CYLINDRICAL_SURFACE ( 'NONE', #3981, 2.500000000000002220 ) ;
#1752=CIRCLE ( 'NONE', #3881, 5.000000000000004441 ) ;
#1754=VECTOR ( 'NONE', #115, 1000.000000000000000 ) ;
#1758=AXIS2_PLACEMENT_3D ( 'NONE', #683, #5330, #2044 ) ;
#1762=CARTESIAN_POINT ( 'NONE',  ( 65.00000000000001421, -1.951563910473909559E-15, 55.00000000000000000 ) ) ;
#1775=DIRECTION ( 'NONE',  ( -0.000000000000000000, -0.000000000000000000, -1.000000000000000000 ) ) ;
#1776=ORIENTED_EDGE ( 'NONE', *, *, #611, .T. ) ;
#1784=ORIENTED_EDGE ( 'NONE', *, *, #5319, .F. ) ;
#1785=CARTESIAN_POINT ( 'NONE',  ( -74.99999999999998579, 15.00000000000000000, 75.00000000000000000 ) ) ;
#1789=DIRECTION ( 'NONE',  ( 0.000000000000000000, -1.734723475976808080E-16, -1.000000000000000000 ) ) ;
#1794=VERTEX_POINT ( 'NONE', #389 ) ;
#1799=PLANE ( 'NONE',  #4574 ) ;
#1814=CARTESIAN_POINT ( 'NONE',  ( 75.00000000000001421, -7.000000000000007105, -75.00000000000000000 ) ) ;
#1816=FACE_OUTER_BOUND ( 'NONE', #2349, .T. ) ;
#1817=DIRECTION ( 'NONE',  ( -0.000000000000000000, -0.000000000000000000, 1.000000000000000000 ) ) ;
#1818=EDGE_LOOP ( 'NONE', ( #1199, #4772, #2611, #1887 ) ) ;
#1823=EDGE_CURVE ( 'NONE', #2749, #2650, #2502, .T. ) ;
#1824=CARTESIAN_POINT ( 'NONE',  ( 37.50000000000000711, 6.288372600415927295E-15, 55.00000000000000000 ) ) ;
#1834=CARTESIAN_POINT ( 'NONE',  ( 25.00000000000000711, -6.999999999999988454, 65.00000000000000000 ) ) ;
#1835=DIRECTION ( 'NONE',  ( 1.000000000000000000, 0.000000000000000000, 0.000000000000000000 ) ) ;
#1836=DIRECTION ( 'NONE',  ( 0.000000000000000000, 0.000000000000000000, -1.000000000000000000 ) ) ;
#1837=CIRCLE ( 'NONE', #874, 0.9999999999999991118 ) ;
#1844=FACE_OUTER_BOUND ( 'NONE', #4281, .T. ) ;
#1846=CARTESIAN_POINT ( 'NONE',  ( 75.00000000000001421, -7.000000000000006217, 65.00000000000000000 ) ) ;
#1848=CARTESIAN_POINT ( 'NONE',  ( 75.00000000000001421, 0.000000000000000000, 8.500000000000000000 ) ) ;
#1849=AXIS2_PLACEMENT_3D ( 'NONE', #5851, #1721, #3744 ) ;
#1850=CIRCLE ( 'NONE', #4965, 0.9999999999999991118 ) ;
#1859=CARTESIAN_POINT ( 'NONE',  ( 65.00000000000001421, -1.951563910473909559E-15, 65.00000000000000000 ) ) ;
#1861=VERTEX_POINT ( 'NONE', #3292 ) ;
#1868=CARTESIAN_POINT ( 'NONE',  ( 75.00000000000001421, -7.000000000000006217, -65.00000000000000000 ) ) ;
#1870=LINE ( 'NONE', #1415, #1993 ) ;
#1872=EDGE_CURVE ( 'NONE', #2273, #695, #2807, .T. ) ;
#1873=FACE_OUTER_BOUND ( 'NONE', #4, .T. ) ;
#1875=VERTEX_POINT ( 'NONE', #4149 ) ;
#1877=EDGE_CURVE ( 'NONE', #5450, #4416, #4698, .T. ) ;
#1886=ORIENTED_EDGE ( 'NONE', *, *, #4664, .F. ) ;
#1887=ORIENTED_EDGE ( 'NONE', *, *, #3941, .T. ) ;
#1899=EDGE_CURVE ( 'NONE', #736, #1175, #476, .T. ) ;
#1902=EDGE_LOOP ( 'NONE', ( #1886, #5125, #1486, #4835 ) ) ;
#1911=ORIENTED_EDGE ( 'NONE', *, *, #3225, .T. ) ;
#1917=LINE ( 'NONE', #1868, #4763 ) ;
#1930=CONICAL_SURFACE ( 'NONE', #5337, 2.500000000000002220, 1.029744260000002631 ) ;
#1934=ORIENTED_EDGE ( 'NONE', *, *, #4765, .T. ) ;
#1935=PLANE ( 'NONE',  #1473 ) ;
#1941=CIRCLE ( 'NONE', #1758, 7.000000000000000000 ) ;
#1957=LINE ( 'NONE', #2415, #4468 ) ;
#1960=EDGE_LOOP ( 'NONE', ( #447, #5955, #2287, #2361, #2096, #4038, #4925, #3541, #1537, #2616, #4884, #1196 ) ) ;
#1969=LINE ( 'NONE', #4804, #1977 ) ;
#1977=VECTOR ( 'NONE', #4715, 1000.000000000000114 ) ;
#1979=EDGE_LOOP ( 'NONE', ( #5834, #4788, #2682, #2573, #4041, #5413, #1784, #2694 ) ) ;
#1980=CARTESIAN_POINT ( 'NONE',  ( 75.00000000000001421, 0.000000000000000000, 9.500000000000000000 ) ) ;
#1981=CARTESIAN_POINT ( 'NONE',  ( 37.50000000000000711, 6.288372600415927295E-15, -65.00000000000000000 ) ) ;
#1982=FACE_OUTER_BOUND ( 'NONE', #3729, .T. ) ;
#1992=EDGE_LOOP ( 'NONE', ( #3694, #4300, #1510 ) ) ;
#1993=VECTOR ( 'NONE', #3837, 1000.000000000000000 ) ;
#2002=ADVANCED_FACE ( 'NONE', ( #3470 ), #4782, .F. ) ;
#2003=VERTEX_POINT ( 'NONE', #4329 ) ;
#2004=LINE ( 'NONE', #1590, #3295 ) ;
#2006=CARTESIAN_POINT ( 'NONE',  ( 37.50000000000000711, 6.288372600415927295E-15, -65.00000000000000000 ) ) ;
#2007=ORIENTED_EDGE ( 'NONE', *, *, #2699, .T. ) ;
#2031=CONICAL_SURFACE ( 'NONE', #1549, 2.500000000000002220, 1.029744260000002631 ) ;
#2032=CARTESIAN_POINT ( 'NONE',  ( 75.00000000000001421, 0.000000000000000000, -7.000000000000000000 ) ) ;
#2041=CIRCLE ( 'NONE', #3596, 2.500000000000002220 ) ;
#2044=DIRECTION ( 'NONE',  ( 0.000000000000000000, 0.000000000000000000, -1.000000000000000000 ) ) ;
#2048=CIRCLE ( 'NONE', #697, 7.000000000000000000 ) ;
#2049=CARTESIAN_POINT ( 'NONE',  ( 25.00000000000000711, -6.999999999999988454, 65.00000000000000000 ) ) ;
#2050=EDGE_CURVE ( 'NONE', #2958, #1875, #3384, .T. ) ;
#2064=LINE ( 'NONE', #5531, #3982 ) ;
#2065=FILL_AREA_STYLE ('',( #4378 ) ) ;
#2071=EDGE_LOOP ( 'NONE', ( #351, #3448 ) ) ;
#2072=CARTESIAN_POINT ( 'NONE',  ( -45.00000000000002842, 15.00000000000000000, -44.99999999999998579 ) ) ;
#2077=VECTOR ( 'NONE', #3878, 1000.000000000000000 ) ;
#2078=CYLINDRICAL_SURFACE ( 'NONE', #5919, 0.9999999999999991118 ) ;
#2086=EDGE_CURVE ( 'NONE', #4227, #3393, #1246, .T. ) ;
#2088=EDGE_CURVE ( 'NONE', #4783, #4354, #5708, .T. ) ;
#2090=CARTESIAN_POINT ( 'NONE',  ( 25.00000000000000711, -6.999999999999988454, -65.00000000000000000 ) ) ;
#2091=PRODUCT_DEFINITION_CONTEXT ( 'detailed design', #555, 'design' ) ;
#2094=LINE ( 'NONE', #732, #5600 ) ;
#2096=ORIENTED_EDGE ( 'NONE', *, *, #3225, .F. ) ;
#2104=DIRECTION ( 'NONE',  ( -0.000000000000000000, -0.000000000000000000, -1.000000000000000000 ) ) ;
#2110=FACE_OUTER_BOUND ( 'NONE', #5956, .T. ) ;
#2119=EDGE_LOOP ( 'NONE', ( #2199, #81, #1911, #2835, #2730, #4075, #4394, #2291 ) ) ;
#2121=( NAMED_UNIT ( * ) SI_UNIT ( $, .STERADIAN. ) SOLID_ANGLE_UNIT ( ) );
#2124=CARTESIAN_POINT ( 'NONE',  ( 55.00000000000000711, 8.572527594031473190E-16, 7.000000000000000000 ) ) ;
#2128=VECTOR ( 'NONE', #4918, 1000.000000000000000 ) ;
#2133=ORIENTED_EDGE ( 'NONE', *, *, #2548, .T. ) ;
#2134=DIRECTION ( 'NONE',  ( 0.000000000000000000, 1.000000000000000000, 0.000000000000000000 ) ) ;
#2138=VECTOR ( 'NONE', #116, 1000.000000000000000 ) ;
#2141=LINE ( 'NONE', #4821, #2128 ) ;
#2146=AXIS2_PLACEMENT_3D ( 'NONE', #1340, #895, #974 ) ;
#2151=EDGE_LOOP ( 'NONE', ( #998, #1254, #357, #5562 ) ) ;
#2161=EDGE_LOOP ( 'NONE', ( #1282, #290, #5181 ) ) ;
#2162=EDGE_CURVE ( 'NONE', #5475, #1708, #801, .T. ) ;
#2165=CARTESIAN_POINT ( 'NONE',  ( 37.50000000000000711, 6.288372600415927295E-15, 65.00000000000000000 ) ) ;
#2167=EDGE_CURVE ( 'NONE', #1426, #5354, #574, .T. ) ;
#2172=ORIENTED_EDGE ( 'NONE', *, *, #1082, .T. ) ;
#2187=DIRECTION ( 'NONE',  ( -0.000000000000000000, -0.000000000000000000, -1.000000000000000000 ) ) ;
#2188=ORIENTED_EDGE ( 'NONE', *, *, #611, .F. ) ;
#2192=ORIENTED_EDGE ( 'NONE', *, *, #2465, .T. ) ;
#2199=ORIENTED_EDGE ( 'NONE', *, *, #2906, .F. ) ;
#2200=ADVANCED_FACE ( 'NONE', ( #855 ), #2258, .F. ) ;
#2202=CARTESIAN_POINT ( 'NONE',  ( 67.00000000000000000, 1.224646799147354440E-16, -8.500000000000000000 ) ) ;
#2208=EDGE_CURVE ( 'NONE', #5930, #554, #5332, .T. ) ;
#2219=ORIENTED_EDGE ( 'NONE', *, *, #3575, .T. ) ;
#2224=CARTESIAN_POINT ( 'NONE',  ( 75.00000000000001421, 8.572527594031473190E-16, 7.000000000000000000 ) ) ;
#2228=VERTEX_POINT ( 'NONE', #1459 ) ;
#2240=DIRECTION ( 'NONE',  ( 0.000000000000000000, 0.000000000000000000, -1.000000000000000000 ) ) ;
#2243=ADVANCED_FACE ( 'NONE', ( #5171 ), #2903, .F. ) ;
#2245=VECTOR ( 'NONE', #4173, 1000.000000000000000 ) ;
#2249=VECTOR ( 'NONE', #568, 1000.000000000000000 ) ;
#2253=ORIENTED_EDGE ( 'NONE', *, *, #2566, .F. ) ;
#2255=FACE_OUTER_BOUND ( 'NONE', #2119, .T. ) ;
#2258=PLANE ( 'NONE',  #4951 ) ;
#2267=CIRCLE ( 'NONE', #5464, 5.000000000000004441 ) ;
#2272=DIRECTION ( 'NONE',  ( 0.000000000000000000, 1.000000000000000000, 0.000000000000000000 ) ) ;
#2273=VERTEX_POINT ( 'NONE', #4717 ) ;
#2281=DIRECTION ( 'NONE',  ( 1.000000000000000000, -0.000000000000000000, -0.000000000000000000 ) ) ;
#2287=ORIENTED_EDGE ( 'NONE', *, *, #315, .T. ) ;
#2291=ORIENTED_EDGE ( 'NONE', *, *, #2458, .F. ) ;
#2292=EDGE_LOOP ( 'NONE', ( #41, #2865, #2774 ) ) ;
#2296=CARTESIAN_POINT ( 'NONE',  ( 67.00000000000000000, 0.000000000000000000, 9.500000000000000000 ) ) ;
#2297=DIRECTION ( 'NONE',  ( 0.000000000000000000, 8.673617379884040402E-17, 1.000000000000000000 ) ) ;
#2301=LINE ( 'NONE', #1046, #34 ) ;
#2302=ADVANCED_FACE ( 'NONE', ( #2857 ), #484, .F. ) ;
#2307=EDGE_CURVE ( 'NONE', #1708, #3671, #3581, .T. ) ;
#2326=DIRECTION ( 'NONE',  ( -1.000000000000000000, 0.000000000000000000, 0.000000000000000000 ) ) ;
#2349=EDGE_LOOP ( 'NONE', ( #3466, #5025, #4899, #1192 ) ) ;
#2356=PLANE ( 'NONE',  #4666 ) ;
#2361=ORIENTED_EDGE ( 'NONE', *, *, #910, .F. ) ;
#2364=EDGE_CURVE ( 'NONE', #782, #4209, #1440, .T. ) ;
#2367=ORIENTED_EDGE ( 'NONE', *, *, #390, .T. ) ;
#2372=LINE ( 'NONE', #3680, #503 ) ;
#2388=CARTESIAN_POINT ( 'NONE',  ( 25.00000000000000711, -6.999999999999989342, -75.00000000000000000 ) ) ;
#2390=VERTEX_POINT ( 'NONE', #2032 ) ;
#2396=DIRECTION ( 'NONE',  ( 0.000000000000000000, 0.000000000000000000, -1.000000000000000000 ) ) ;
#2399=CARTESIAN_POINT ( 'NONE',  ( 37.50000000000000711, 6.288372600415927295E-15, -55.00000000000000000 ) ) ;
#2407=DIRECTION ( 'NONE',  ( 1.000000000000000000, 0.000000000000000000, -0.000000000000000000 ) ) ;
#2409=VECTOR ( 'NONE', #2584, 1000.000000000000000 ) ;
#2415=CARTESIAN_POINT ( 'NONE',  ( 60.00000000000001421, -1.645402210687070900E-15, 65.00000000000000000 ) ) ;
#2428=EDGE_LOOP ( 'NONE', ( #444, #4136 ) ) ;
#2436=VERTEX_POINT ( 'NONE', #3439 ) ;
#2440=VERTEX_POINT ( 'NONE', #2887 ) ;
#2446=DIRECTION ( 'NONE',  ( 0.000000000000000000, 0.000000000000000000, -1.000000000000000000 ) ) ;
#2451=ORIENTED_EDGE ( 'NONE', *, *, #2162, .F. ) ;
#2458=EDGE_CURVE ( 'NONE', #1041, #695, #2952, .T. ) ;
#2464=ORIENTED_EDGE ( 'NONE', *, *, #5604, .F. ) ;
#2465=EDGE_CURVE ( 'NONE', #360, #554, #5645, .T. ) ;
#2467=CARTESIAN_POINT ( 'NONE',  ( 25.00000000000000711, -6.999999999999988454, 65.00000000000000000 ) ) ;
#2474=CARTESIAN_POINT ( 'NONE',  ( -45.00000000000002842, 0.000000000000000000, -44.99999999999998579 ) ) ;
#2480=VECTOR ( 'NONE', #1091, 1000.000000000000000 ) ;
#2487=EDGE_LOOP ( 'NONE', ( #5907, #3232, #1128, #3539 ) ) ;
#2498=DIRECTION ( 'NONE',  ( -0.000000000000000000, -0.000000000000000000, -1.000000000000000000 ) ) ;
#2502=CIRCLE ( 'NONE', #4261, 0.9999999999999991118 ) ;
#2504=EDGE_CURVE ( 'NONE', #2228, #5607, #4176, .T. ) ;
#2508=AXIS2_PLACEMENT_3D ( 'NONE', #4379, #312, #1121 ) ;
#2509=EDGE_LOOP ( 'NONE', ( #4749, #2007, #2624 ) ) ;
#2518=CIRCLE ( 'NONE', #1849, 5.000000000000004441 ) ;
#2519=VECTOR ( 'NONE', #1069, 1000.000000000000000 ) ;
#2523=VERTEX_POINT ( 'NONE', #3073 ) ;
#2525=CIRCLE ( 'NONE', #3228, 0.9999999999999991118 ) ;
#2532=ORIENTED_EDGE ( 'NONE', *, *, #826, .T. ) ;
#2535=EDGE_CURVE ( 'NONE', #1175, #4444, #4996, .T. ) ;
#2543=ORIENTED_EDGE ( 'NONE', *, *, #753, .T. ) ;
#2547=FACE_BOUND ( 'NONE', #4417, .T. ) ;
#2548=EDGE_CURVE ( 'NONE', #360, #5930, #5858, .T. ) ;
#2550=( LENGTH_UNIT ( ) NAMED_UNIT ( * ) SI_UNIT ( .MILLI., .METRE. ) );
#2551=LINE ( 'NONE', #4413, #3965 ) ;
#2562=DIRECTION ( 'NONE',  ( 0.000000000000000000, 0.000000000000000000, -1.000000000000000000 ) ) ;
#2566=EDGE_CURVE ( 'NONE', #5507, #3782, #1730, .T. ) ;
#2568=DIRECTION ( 'NONE',  ( -0.000000000000000000, -0.000000000000000000, 1.000000000000000000 ) ) ;
#2573=ORIENTED_EDGE ( 'NONE', *, *, #2088, .F. ) ;
#2577=( NAMED_UNIT ( * ) PLANE_ANGLE_UNIT ( ) SI_UNIT ( $, .RADIAN. ) );
#2582=ORIENTED_EDGE ( 'NONE', *, *, #2167, .T. ) ;
#2584=DIRECTION ( 'NONE',  ( -0.8571673013836870192, 1.049727191973306873E-16, 0.5150380737757234151 ) ) ;
#2587=CARTESIAN_POINT ( 'NONE',  ( 62.50000000000001421, -1.951563910473909559E-15, -55.00000000000000000 ) ) ;
#2589=LINE ( 'NONE', #4452, #5827 ) ;
#2604=EDGE_CURVE ( 'NONE', #1794, #3819, #851, .T. ) ;
#2611=ORIENTED_EDGE ( 'NONE', *, *, #5498, .T. ) ;
#2612=ORIENTED_EDGE ( 'NONE', *, *, #224, .T. ) ;
#2616=ORIENTED_EDGE ( 'NONE', *, *, #4653, .T. ) ;
#2624=ORIENTED_EDGE ( 'NONE', *, *, #1348, .T. ) ;
#2627=AXIS2_PLACEMENT_3D ( 'NONE', #3595, #2104, #835 ) ;
#2630=DIRECTION ( 'NONE',  ( 0.000000000000000000, 0.000000000000000000, -1.000000000000000000 ) ) ;
#2633=AXIS2_PLACEMENT_3D ( 'NONE', #5358, #4906, #352 ) ;
#2635=CIRCLE ( 'NONE', #4084, 5.000000000000004441 ) ;
#2643=DIRECTION ( 'NONE',  ( -1.000000000000000000, 0.000000000000000000, 0.000000000000000000 ) ) ;
#2646=CARTESIAN_POINT ( 'NONE',  ( 37.50000000000000711, 6.288372600415927295E-15, -55.00000000000000000 ) ) ;
#2650=VERTEX_POINT ( 'NONE', #3166 ) ;
#2657=DIRECTION ( 'NONE',  ( -0.000000000000000000, -0.000000000000000000, -1.000000000000000000 ) ) ;
#2659=DIRECTION ( 'NONE',  ( -1.000000000000000000, -0.000000000000000000, -0.000000000000000000 ) ) ;
#2660=ORIENTED_EDGE ( 'NONE', *, *, #5731, .F. ) ;
#2662=EDGE_CURVE ( 'NONE', #4209, #2523, #1957, .T. ) ;
#2667=ORIENTED_EDGE ( 'NONE', *, *, #876, .F. ) ;
#2678=VERTEX_POINT ( 'NONE', #4103 ) ;
#2679=CARTESIAN_POINT ( 'NONE',  ( 25.00000000000000711, -6.999999999999988454, -65.00000000000000000 ) ) ;
#2680=CARTESIAN_POINT ( 'NONE',  ( -45.00000000000001421, 15.00000000000000000, 45.00000000000000000 ) ) ;
#2682=ORIENTED_EDGE ( 'NONE', *, *, #2764, .T. ) ;
#2684=EDGE_CURVE ( 'NONE', #2958, #2749, #3839, .T. ) ;
#2694=ORIENTED_EDGE ( 'NONE', *, *, #315, .F. ) ;
#2698=PLANE ( 'NONE',  #5162 ) ;
#2699=EDGE_CURVE ( 'NONE', #4855, #5607, #1044, .T. ) ;
#2710=LINE ( 'NONE', #4609, #5539 ) ;
#2712=CARTESIAN_POINT ( 'NONE',  ( 25.00000000000000711, 7.000000000000009770, 75.00000000000000000 ) ) ;
#2724=ORIENTED_EDGE ( 'NONE', *, *, #4765, .F. ) ;
#2730=ORIENTED_EDGE ( 'NONE', *, *, #141, .T. ) ;
#2731=VECTOR ( 'NONE', #3055, 1000.000000000000000 ) ;
#2732=FACE_BOUND ( 'NONE', #4315, .T. ) ;
#2737=DIRECTION ( 'NONE',  ( -1.000000000000000000, 0.000000000000000000, 0.000000000000000000 ) ) ;
#2740=AXIS2_PLACEMENT_3D ( 'NONE', #3813, #3276, #5128 ) ;
#2748=DIRECTION ( 'NONE',  ( 1.000000000000000000, 0.000000000000000000, 0.000000000000000000 ) ) ;
#2749=VERTEX_POINT ( 'NONE', #151 ) ;
#2757=CARTESIAN_POINT ( 'NONE',  ( 62.50000000000001421, -1.951563910473909559E-15, 55.00000000000000000 ) ) ;
#2763=CARTESIAN_POINT ( 'NONE',  ( 75.00000000000001421, -15.00000000000000355, 75.00000000000000000 ) ) ;
#2764=EDGE_CURVE ( 'NONE', #3819, #4354, #5186, .T. ) ;
#2768=ORIENTED_EDGE ( 'NONE', *, *, #4653, .F. ) ;
#2774=ORIENTED_EDGE ( 'NONE', *, *, #4664, .T. ) ;
#2787=CARTESIAN_POINT ( 'NONE',  ( -74.99999999999998579, -15.00000000000000000, 75.00000000000000000 ) ) ;
#2794=ORIENTED_EDGE ( 'NONE', *, *, #141, .F. ) ;
#2797=DIRECTION ( 'NONE',  ( 0.000000000000000000, 1.000000000000000000, 0.000000000000000000 ) ) ;
#2798=DIRECTION ( 'NONE',  ( 0.000000000000000000, 0.000000000000000000, 1.000000000000000000 ) ) ;
#2806=ADVANCED_FACE ( 'NONE', ( #2110 ), #4340, .F. ) ;
#2807=LINE ( 'NONE', #5971, #3286 ) ;
#2811=VECTOR ( 'NONE', #4443, 1000.000000000000000 ) ;
#2815=AXIS2_PLACEMENT_3D ( 'NONE', #2959, #262, #2987 ) ;
#2821=CYLINDRICAL_SURFACE ( 'NONE', #3128, 2.500000000000002220 ) ;
#2822=VECTOR ( 'NONE', #2659, 1000.000000000000000 ) ;
#2828=LINE ( 'NONE', #759, #3935 ) ;
#2829=ADVANCED_FACE ( 'NONE', ( #3030 ), #1930, .F. ) ;
#2835=ORIENTED_EDGE ( 'NONE', *, *, #3907, .T. ) ;
#2836=PLANE ( 'NONE',  #399 ) ;
#2850=EDGE_LOOP ( 'NONE', ( #728, #2133, #1397 ) ) ;
#2854=CARTESIAN_POINT ( 'NONE',  ( 62.50000000000001421, -1.951563910473909559E-15, 55.00000000000000000 ) ) ;
#2857=FACE_OUTER_BOUND ( 'NONE', #2509, .T. ) ;
#2861=FACE_OUTER_BOUND ( 'NONE', #1240, .T. ) ;
#2865=ORIENTED_EDGE ( 'NONE', *, *, #4106, .T. ) ;
#2866=CARTESIAN_POINT ( 'NONE',  ( 67.00000000000000000, 0.000000000000000000, -10.49999999999999822 ) ) ;
#2868=DIRECTION ( 'NONE',  ( 1.000000000000000000, 0.000000000000000000, 0.000000000000000000 ) ) ;
#2870=AXIS2_PLACEMENT_3D ( 'NONE', #5127, #958, #2446 ) ;
#2879=DIRECTION ( 'NONE',  ( 0.000000000000000000, 1.000000000000000000, 0.000000000000000000 ) ) ;
#2884=DIRECTION ( 'NONE',  ( 0.000000000000000000, -1.000000000000000000, 0.000000000000000000 ) ) ;
#2887=CARTESIAN_POINT ( 'NONE',  ( 75.00000000000001421, 15.00000000000000000, -75.00000000000000000 ) ) ;
#2890=ORIENTED_EDGE ( 'NONE', *, *, #1823, .T. ) ;
#2891=DIRECTION ( 'NONE',  ( -0.000000000000000000, -0.000000000000000000, -1.000000000000000000 ) ) ;
#2892=DIRECTION ( 'NONE',  ( -1.000000000000000000, 0.000000000000000000, 0.000000000000000000 ) ) ;
#2899=EDGE_CURVE ( 'NONE', #4444, #3189, #582, .T. ) ;
#2903=CONICAL_SURFACE ( 'NONE', #774, 2.500000000000002220, 1.029744260000002631 ) ;
#2905=CARTESIAN_POINT ( 'NONE',  ( 75.00000000000001421, 0.000000000000000000, -10.49999999999999822 ) ) ;
#2906=EDGE_CURVE ( 'NONE', #2003, #1041, #2141, .T. ) ;
#2908=ORIENTED_EDGE ( 'NONE', *, *, #3785, .T. ) ;
#2911=LINE ( 'NONE', #5698, #4108 ) ;
#2914=ADVANCED_FACE ( 'NONE', ( #299 ), #5148, .F. ) ;
#2919=AXIS2_PLACEMENT_3D ( 'NONE', #2679, #380, #4018 ) ;
#2927=VECTOR ( 'NONE', #1169, 1000.000000000000000 ) ;
#2929=DIRECTION ( 'NONE',  ( -0.000000000000000000, -0.000000000000000000, -1.000000000000000000 ) ) ;
#2930=EDGE_LOOP ( 'NONE', ( #1934, #1333, #807, #3815 ) ) ;
#2935=( GEOMETRIC_REPRESENTATION_CONTEXT ( 3 ) GLOBAL_UNCERTAINTY_ASSIGNED_CONTEXT ( ( #5251 ) ) GLOBAL_UNIT_ASSIGNED_CONTEXT ( ( #4802, #227, #1182 ) ) REPRESENTATION_CONTEXT ( 'NONE', 'WORKASPACE' ) );
#2942=EDGE_LOOP ( 'NONE', ( #344, #2964, #1112, #2667 ) ) ;
#2950=ADVANCED_FACE ( 'NONE', ( #2996 ), #3479, .F. ) ;
#2952=LINE ( 'NONE', #5292, #3969 ) ;
#2958=VERTEX_POINT ( 'NONE', #2202 ) ;
#2959=CARTESIAN_POINT ( 'NONE',  ( 75.00000000000001421, 0.000000000000000000, -9.500000000000000000 ) ) ;
#2964=ORIENTED_EDGE ( 'NONE', *, *, #5599, .T. ) ;
#2967=CARTESIAN_POINT ( 'NONE',  ( 75.00000000000001421, 0.000000000000000000, 9.500000000000000000 ) ) ;
#2969=CIRCLE ( 'NONE', #3359, 2.500000000000002220 ) ;
#2982=EDGE_LOOP ( 'NONE', ( #524, #589, #4632 ) ) ;
#2984=DIRECTION ( 'NONE',  ( 1.000000000000000000, -3.469446951953614189E-16, 0.000000000000000000 ) ) ;
#2985=CARTESIAN_POINT ( 'NONE',  ( 67.00000000000000000, 0.000000000000000000, -9.500000000000000000 ) ) ;
#2986=ORIENTED_EDGE ( 'NONE', *, *, #5234, .T. ) ;
#2987=DIRECTION ( 'NONE',  ( 0.000000000000000000, 0.000000000000000000, -1.000000000000000000 ) ) ;
#2989=CARTESIAN_POINT ( 'NONE',  ( 67.00000000000000000, 0.000000000000000000, 9.500000000000000000 ) ) ;
#2996=FACE_OUTER_BOUND ( 'NONE', #929, .T. ) ;
#2998=DIRECTION ( 'NONE',  ( -1.000000000000000000, 0.000000000000000000, 0.000000000000000000 ) ) ;
#3008=DIRECTION ( 'NONE',  ( 0.000000000000000000, -1.000000000000000000, 0.000000000000000000 ) ) ;
#3030=FACE_OUTER_BOUND ( 'NONE', #2982, .T. ) ;
#3034=ADVANCED_FACE ( 'NONE', ( #1261 ), #4180, .F. ) ;
#3049=ORIENTED_EDGE ( 'NONE', *, *, #1877, .T. ) ;
#3052=DIRECTION ( 'NONE',  ( 0.000000000000000000, 0.000000000000000000, -1.000000000000000000 ) ) ;
#3053=DIRECTION ( 'NONE',  ( -1.000000000000000000, 0.000000000000000000, 0.000000000000000000 ) ) ;
#3055=DIRECTION ( 'NONE',  ( -0.000000000000000000, -0.000000000000000000, -1.000000000000000000 ) ) ;
#3061=DIRECTION ( 'NONE',  ( 0.000000000000000000, 0.000000000000000000, -1.000000000000000000 ) ) ;
#3063=CARTESIAN_POINT ( 'NONE',  ( 37.50000000000000711, 6.288372600415927295E-15, 65.00000000000000000 ) ) ;
#3065=EDGE_CURVE ( 'NONE', #5793, #2003, #5041, .T. ) ;
#3066=CARTESIAN_POINT ( 'NONE',  ( 25.00000000000000711, 7.000000000000009770, -75.00000000000000000 ) ) ;
#3071=CONICAL_SURFACE ( 'NONE', #1221, 2.500000000000002220, 1.029744260000002631 ) ;
#3073=CARTESIAN_POINT ( 'NONE',  ( 60.00000000000001421, -1.645402210687070900E-15, 65.00000000000000000 ) ) ;
#3074=ORIENTED_EDGE ( 'NONE', *, *, #5835, .F. ) ;
#3082=CARTESIAN_POINT ( 'NONE',  ( 60.00000000000001421, -1.951563910473909559E-15, -55.00000000000000000 ) ) ;
#3088=CARTESIAN_POINT ( 'NONE',  ( -74.99999999999998579, -15.00000000000000000, -75.00000000000000000 ) ) ;
#3104=EDGE_CURVE ( 'NONE', #5094, #1875, #4181, .T. ) ;
#3125=AXIS2_PLACEMENT_3D ( 'NONE', #5938, #1205, #3603 ) ;
#3128=AXIS2_PLACEMENT_3D ( 'NONE', #572, #5192, #1002 ) ;
#3129=VECTOR ( 'NONE', #3172, 1000.000000000000000 ) ;
#3134=VECTOR ( 'NONE', #2797, 1000.000000000000000 ) ;
#3140=LINE ( 'NONE', #1369, #730 ) ;
#3143=DIRECTION ( 'NONE',  ( -0.000000000000000000, -0.000000000000000000, 1.000000000000000000 ) ) ;
#3144=VECTOR ( 'NONE', #1209, 1000.000000000000000 ) ;
#3149=FACE_OUTER_BOUND ( 'NONE', #2942, .T. ) ;
#3153=LINE ( 'NONE', #5472, #3134 ) ;
#3161=PLANE ( 'NONE',  #4328 ) ;
#3166=CARTESIAN_POINT ( 'NONE',  ( 75.00000000000001421, 0.000000000000000000, -10.49999999999999822 ) ) ;
#3172=DIRECTION ( 'NONE',  ( 0.000000000000000000, -1.734723475976808080E-16, -1.000000000000000000 ) ) ;
#3181=DIRECTION ( 'NONE',  ( 0.000000000000000000, 0.000000000000000000, -1.000000000000000000 ) ) ;
#3188=DIRECTION ( 'NONE',  ( 0.000000000000000000, -1.000000000000000000, 0.000000000000000000 ) ) ;
#3189=VERTEX_POINT ( 'NONE', #56 ) ;
#3193=ORIENTED_EDGE ( 'NONE', *, *, #824, .T. ) ;
#3194=FACE_OUTER_BOUND ( 'NONE', #535, .T. ) ;
#3196=LINE ( 'NONE', #1762, #4557 ) ;
#3204=CARTESIAN_POINT ( 'NONE',  ( 37.50000000000000711, 6.288372600415927295E-15, 55.00000000000000000 ) ) ;
#3205=VERTEX_POINT ( 'NONE', #1498 ) ;
#3218=DIRECTION ( 'NONE',  ( 1.000000000000000000, 0.000000000000000000, 0.000000000000000000 ) ) ;
#3221=AXIS2_PLACEMENT_3D ( 'NONE', #1536, #3188, #5043 ) ;
#3225=EDGE_CURVE ( 'NONE', #3927, #5326, #592, .T. ) ;
#3228=AXIS2_PLACEMENT_3D ( 'NONE', #4450, #328, #3990 ) ;
#3232=ORIENTED_EDGE ( 'NONE', *, *, #4511, .F. ) ;
#3245=CARTESIAN_POINT ( 'NONE',  ( 75.00000000000001421, -15.00000000000000355, 75.00000000000000000 ) ) ;
#3246=CARTESIAN_POINT ( 'NONE',  ( 75.00000000000001421, 1.224646799147353207E-16, 10.49999999999999822 ) ) ;
#3247=ORIENTED_EDGE ( 'NONE', *, *, #224, .F. ) ;
#3260=LINE ( 'NONE', #4652, #3129 ) ;
#3263=FACE_OUTER_BOUND ( 'NONE', #2850, .T. ) ;
#3265=ORIENTED_EDGE ( 'NONE', *, *, #2208, .F. ) ;
#3267=DIRECTION ( 'NONE',  ( 0.000000000000000000, -0.000000000000000000, -1.000000000000000000 ) ) ;
#3276=DIRECTION ( 'NONE',  ( 0.000000000000000000, 1.000000000000000000, 0.000000000000000000 ) ) ;
#3277=EDGE_CURVE ( 'NONE', #4209, #782, #5911, .T. ) ;
#3279=DIRECTION ( 'NONE',  ( -0.000000000000000000, -0.000000000000000000, -1.000000000000000000 ) ) ;
#3282=DIRECTION ( 'NONE',  ( 1.000000000000000000, -0.000000000000000000, -0.000000000000000000 ) ) ;
#3285=ORIENTED_EDGE ( 'NONE', *, *, #5301, .F. ) ;
#3286=VECTOR ( 'NONE', #5151, 1000.000000000000000 ) ;
#3292=CARTESIAN_POINT ( 'NONE',  ( -45.00000000000001421, 0.000000000000000000, 50.00000000000000000 ) ) ;
#3295=VECTOR ( 'NONE', #4327, 1000.000000000000000 ) ;
#3298=AXIS2_PLACEMENT_3D ( 'NONE', #723, #246, #1570 ) ;
#3310=VECTOR ( 'NONE', #2657, 1000.000000000000000 ) ;
#3314=CARTESIAN_POINT ( 'NONE',  ( -45.00000000000001421, 15.00000000000000000, 39.99999999999999289 ) ) ;
#3316=ADVANCED_FACE ( 'NONE', ( #680 ), #740, .F. ) ;
#3323=ORIENTED_EDGE ( 'NONE', *, *, #3065, .T. ) ;
#3335=ADVANCED_FACE ( 'NONE', ( #1129 ), #5270, .F. ) ;
#3343=EDGE_LOOP ( 'NONE', ( #1291, #1224, #2253, #5061 ) ) ;
#3359=AXIS2_PLACEMENT_3D ( 'NONE', #5103, #4246, #2326 ) ;
#3360=EDGE_LOOP ( 'NONE', ( #3559, #3666 ) ) ;
#3363=CARTESIAN_POINT ( 'NONE',  ( 75.00000000000001421, 1.224646799147353207E-16, -8.500000000000000000 ) ) ;
#3364=CARTESIAN_POINT ( 'NONE',  ( 75.00000000000001421, 0.000000000000000000, 8.500000000000000000 ) ) ;
#3366=ADVANCED_FACE ( 'NONE', ( #5228, #1068, #5806 ), #4784, .F. ) ;
#3375=ORIENTED_EDGE ( 'NONE', *, *, #3998, .F. ) ;
#3384=CIRCLE ( 'NONE', #1732, 0.9999999999999991118 ) ;
#3387=EDGE_CURVE ( 'NONE', #5402, #726, #4860, .T. ) ;
#3393=VERTEX_POINT ( 'NONE', #5685 ) ;
#3395=VECTOR ( 'NONE', #1281, 1000.000000000000000 ) ;
#3396=CARTESIAN_POINT ( 'NONE',  ( -45.00000000000001421, 0.000000000000000000, 45.00000000000000000 ) ) ;
#3399=AXIS2_PLACEMENT_3D ( 'NONE', #1623, #4879, #1157 ) ;
#3400=SHAPE_REPRESENTATION_RELATIONSHIP ( 'NONE' , 'NONE' ,  #5269, #1232 ) ;
#3402=CONICAL_SURFACE ( 'NONE', #4284, 0.9999999999999991118, 1.029744260000008405 ) ;
#3406=VERTEX_POINT ( 'NONE', #5411 ) ;
#3407=AXIS2_PLACEMENT_3D ( 'NONE', #2680, #1158, #4540 ) ;
#3410=VECTOR ( 'NONE', #1789, 1000.000000000000000 ) ;
#3411=AXIS2_PLACEMENT_3D ( 'NONE', #1720, #365, #3636 ) ;
#3437=PLANE ( 'NONE',  #2508 ) ;
#3439=CARTESIAN_POINT ( 'NONE',  ( 75.00000000000001421, 6.999999999999992006, -75.00000000000000000 ) ) ;
#3441=ADVANCED_FACE ( 'NONE', ( #5928 ), #4076, .F. ) ;
#3442=ORIENTED_EDGE ( 'NONE', *, *, #2899, .F. ) ;
#3448=ORIENTED_EDGE ( 'NONE', *, *, #4856, .F. ) ;
#3455=ORIENTED_EDGE ( 'NONE', *, *, #390, .F. ) ;
#3459=CARTESIAN_POINT ( 'NONE',  ( -74.99999999999998579, 15.00000000000000000, 75.00000000000000000 ) ) ;
#3466=ORIENTED_EDGE ( 'NONE', *, *, #3277, .F. ) ;
#3467=ORIENTED_EDGE ( 'NONE', *, *, #39, .F. ) ;
#3470=FACE_OUTER_BOUND ( 'NONE', #1009, .T. ) ;
#3479=CYLINDRICAL_SURFACE ( 'NONE', #684, 0.9999999999999991118 ) ;
#3480=CARTESIAN_POINT ( 'NONE',  ( 25.00000000000000711, -6.999999999999988454, -65.00000000000000000 ) ) ;
#3486=DIRECTION ( 'NONE',  ( 0.000000000000000000, 8.673617379884040402E-17, 1.000000000000000000 ) ) ;
#3488=ORIENTED_EDGE ( 'NONE', *, *, #5137, .T. ) ;
#3500=ADVANCED_FACE ( 'NONE', ( #5960 ), #1799, .F. ) ;
#3519=ORIENTED_EDGE ( 'NONE', *, *, #528, .T. ) ;
#3522=CARTESIAN_POINT ( 'NONE',  ( 25.00000000000000711, -6.999999999999989342, 75.00000000000000000 ) ) ;
#3527=CARTESIAN_POINT ( 'NONE',  ( 0.000000000000000000, 0.000000000000000000, 0.000000000000000000 ) ) ;
#3534=CLOSED_SHELL ( 'NONE', ( #5204, #23, #5947, #3335, #1270, #2302, #2806, #201, #4761, #2829, #4846, #459, #831, #70, #4707, #4355, #1275, #3500, #3316, #311, #372, #5961, #3366, #168, #646, #4955, #1024, #3441, #4997, #208, #61, #4022, #4336, #1084, #3034, #2002, #2243, #254, #4526, #3615, #2914, #5870, #2200, #5208, #1210, #2950, #4097 ) ) ;
#3539=ORIENTED_EDGE ( 'NONE', *, *, #971, .T. ) ;
#3541=ORIENTED_EDGE ( 'NONE', *, *, #694, .F. ) ;
#3542=SHAPE_DEFINITION_REPRESENTATION ( #5189, #5269 ) ;
#3546=CARTESIAN_POINT ( 'NONE',  ( 37.50000000000000711, 6.288372600415927295E-15, -55.00000000000000000 ) ) ;
#3550=DIRECTION ( 'NONE',  ( -0.000000000000000000, -0.000000000000000000, 1.000000000000000000 ) ) ;
#3557=CARTESIAN_POINT ( 'NONE',  ( -45.00000000000002842, 15.00000000000000000, -39.99999999999997868 ) ) ;
#3559=ORIENTED_EDGE ( 'NONE', *, *, #3387, .F. ) ;
#3560=VERTEX_POINT ( 'NONE', #5092 ) ;
#3563=ORIENTED_EDGE ( 'NONE', *, *, #55, .T. ) ;
#3567=DIRECTION ( 'NONE',  ( 1.000000000000000000, -0.000000000000000000, -0.000000000000000000 ) ) ;
#3572=FACE_OUTER_BOUND ( 'NONE', #368, .T. ) ;
#3575=EDGE_CURVE ( 'NONE', #736, #3189, #2064, .T. ) ;
#3576=CARTESIAN_POINT ( 'NONE',  ( 67.00000000000000000, 0.000000000000000000, -9.500000000000000000 ) ) ;
#3581=CIRCLE ( 'NONE', #1054, 2.500000000000002220 ) ;
#3582=EDGE_CURVE ( 'NONE', #1576, #2523, #5434, .T. ) ;
#3592=CARTESIAN_POINT ( 'NONE',  ( 75.00000000000001421, 6.999999999999992006, 75.00000000000000000 ) ) ;
#3595=CARTESIAN_POINT ( 'NONE',  ( 62.50000000000001421, -1.951563910473909559E-15, -65.00000000000000000 ) ) ;
#3596=AXIS2_PLACEMENT_3D ( 'NONE', #1981, #3831, #5302 ) ;
#3598=DIRECTION ( 'NONE',  ( 1.000000000000000000, -0.000000000000000000, -0.000000000000000000 ) ) ;
#3603=DIRECTION ( 'NONE',  ( 0.000000000000000000, 0.000000000000000000, 1.000000000000000000 ) ) ;
#3609=STYLED_ITEM ( 'NONE', ( #4441 ), #1232 ) ;
#3610=CONICAL_SURFACE ( 'NONE', #4092, 2.500000000000002220, 1.029744260000002631 ) ;
#3615=ADVANCED_FACE ( 'NONE', ( #5336 ), #268, .F. ) ;
#3623=PLANE ( 'NONE',  #1579 ) ;
#3636=DIRECTION ( 'NONE',  ( 1.000000000000000000, 0.000000000000000000, 0.000000000000000000 ) ) ;
#3650=CARTESIAN_POINT ( 'NONE',  ( 0.000000000000000000, 0.000000000000000000, 75.00000000000000000 ) ) ;
#3652=DIRECTION ( 'NONE',  ( -1.000000000000000000, 0.000000000000000000, 0.000000000000000000 ) ) ;
#3664=DIRECTION ( 'NONE',  ( -0.000000000000000000, -0.000000000000000000, 1.000000000000000000 ) ) ;
#3666=ORIENTED_EDGE ( 'NONE', *, *, #3706, .F. ) ;
#3671=VERTEX_POINT ( 'NONE', #4339 ) ;
#3675=PRODUCT_CONTEXT ( 'NONE', #5027, 'mechanical' ) ;
#3679=DIRECTION ( 'NONE',  ( 0.000000000000000000, -1.000000000000000000, 0.000000000000000000 ) ) ;
#3680=CARTESIAN_POINT ( 'NONE',  ( 35.00000000000000000, 6.288372600415927295E-15, -55.00000000000000000 ) ) ;
#3685=AXIS2_PLACEMENT_3D ( 'NONE', #2646, #2187, #4961 ) ;
#3694=ORIENTED_EDGE ( 'NONE', *, *, #1389, .F. ) ;
#3697=AXIS2_PLACEMENT_3D ( 'NONE', #1980, #5710, #3830 ) ;
#3700=DIRECTION ( 'NONE',  ( -0.000000000000000000, -0.000000000000000000, -1.000000000000000000 ) ) ;
#3706=EDGE_CURVE ( 'NONE', #726, #5402, #1850, .T. ) ;
#3709=CARTESIAN_POINT ( 'NONE',  ( 0.000000000000000000, 0.000000000000000000, -75.00000000000000000 ) ) ;
#3713=ORIENTED_EDGE ( 'NONE', *, *, #3902, .F. ) ;
#3719=DIRECTION ( 'NONE',  ( 0.000000000000000000, 0.000000000000000000, -1.000000000000000000 ) ) ;
#3727=CARTESIAN_POINT ( 'NONE',  ( -74.99999999999998579, -15.00000000000000000, 75.00000000000000000 ) ) ;
#3729=EDGE_LOOP ( 'NONE', ( #5626, #2192, #1589 ) ) ;
#3741=CARTESIAN_POINT ( 'NONE',  ( 75.00000000000001421, 0.000000000000000000, -9.500000000000000000 ) ) ;
#3744=DIRECTION ( 'NONE',  ( 0.000000000000000000, 0.000000000000000000, -1.000000000000000000 ) ) ;
#3760=CARTESIAN_POINT ( 'NONE',  ( 40.00000000000000711, 6.594534300202765954E-15, -65.00000000000000000 ) ) ;
#3762=EDGE_CURVE ( 'NONE', #3393, #4227, #2041, .T. ) ;
#3776=VECTOR ( 'NONE', #1231, 1000.000000000000000 ) ;
#3782=VERTEX_POINT ( 'NONE', #4785 ) ;
#3785=EDGE_CURVE ( 'NONE', #1708, #1426, #5686, .T. ) ;
#3788=EDGE_CURVE ( 'NONE', #5323, #5481, #237, .T. ) ;
#3805=DIRECTION ( 'NONE',  ( 0.000000000000000000, 0.000000000000000000, -1.000000000000000000 ) ) ;
#3813=CARTESIAN_POINT ( 'NONE',  ( -45.00000000000001421, 0.000000000000000000, 45.00000000000000000 ) ) ;
#3815=ORIENTED_EDGE ( 'NONE', *, *, #5912, .F. ) ;
#3819=VERTEX_POINT ( 'NONE', #4269 ) ;
#3821=CARTESIAN_POINT ( 'NONE',  ( 62.50000000000001421, -1.951563910473909559E-15, 53.49784845693390167 ) ) ;
#3825=ORIENTED_EDGE ( 'NONE', *, *, #4438, .T. ) ;
#3830=DIRECTION ( 'NONE',  ( 0.000000000000000000, 0.000000000000000000, -1.000000000000000000 ) ) ;
#3831=DIRECTION ( 'NONE',  ( -0.000000000000000000, -0.000000000000000000, -1.000000000000000000 ) ) ;
#3834=ORIENTED_EDGE ( 'NONE', *, *, #3785, .F. ) ;
#3837=DIRECTION ( 'NONE',  ( -0.8571673013836870192, 1.049727191973306873E-16, 0.5150380737757234151 ) ) ;
#3839=LINE ( 'NONE', #3363, #4068 ) ;
#3841=CARTESIAN_POINT ( 'NONE',  ( 40.00000000000000711, 6.288372600415927295E-15, 55.00000000000000000 ) ) ;
#3843=ORIENTED_EDGE ( 'NONE', *, *, #3941, .F. ) ;
#3858=EDGE_LOOP ( 'NONE', ( #4639, #1423, #3519, #3825 ) ) ;
#3862=EDGE_CURVE ( 'NONE', #3205, #4999, #2048, .T. ) ;
#3868=CARTESIAN_POINT ( 'NONE',  ( 37.50000000000000711, 6.288372600415927295E-15, -65.00000000000000000 ) ) ;
#3873=LINE ( 'NONE', #4893, #1672 ) ;
#3878=DIRECTION ( 'NONE',  ( -0.000000000000000000, -0.000000000000000000, -1.000000000000000000 ) ) ;
#3881=AXIS2_PLACEMENT_3D ( 'NONE', #4053, #2272, #1235 ) ;
#3883=SURFACE_STYLE_FILL_AREA ( #2065 ) ;
#3888=DIRECTION ( 'NONE',  ( 1.000000000000000000, -3.469446951953614189E-16, -0.000000000000000000 ) ) ;
#3895=ORIENTED_EDGE ( 'NONE', *, *, #4507, .F. ) ;
#3902=EDGE_CURVE ( 'NONE', #1345, #702, #1685, .T. ) ;
#3906=CARTESIAN_POINT ( 'NONE',  ( 60.00000000000001421, -1.951563910473909559E-15, -65.00000000000000000 ) ) ;
#3907=EDGE_CURVE ( 'NONE', #5326, #5390, #5447, .T. ) ;
#3912=LINE ( 'NONE', #3459, #2077 ) ;
#3926=DIRECTION ( 'NONE',  ( 1.000000000000000000, -0.000000000000000000, -0.000000000000000000 ) ) ;
#3927=VERTEX_POINT ( 'NONE', #3592 ) ;
#3935=VECTOR ( 'NONE', #3008, 1000.000000000000000 ) ;
#3941=EDGE_CURVE ( 'NONE', #2650, #2749, #2525, .T. ) ;
#3946=DIRECTION ( 'NONE',  ( 0.5150380737757185301, 1.049727191973310571E-16, 0.8571673013836900168 ) ) ;
#3947=ORIENTED_EDGE ( 'NONE', *, *, #5301, .T. ) ;
#3952=CARTESIAN_POINT ( 'NONE',  ( -74.99999999999998579, -15.00000000000000000, 75.00000000000000000 ) ) ;
#3960=CARTESIAN_POINT ( 'NONE',  ( 37.50000000000000711, 6.288372600415927295E-15, 55.00000000000000000 ) ) ;
#3962=DIRECTION ( 'NONE',  ( -0.000000000000000000, -0.000000000000000000, -1.000000000000000000 ) ) ;
#3965=VECTOR ( 'NONE', #4832, 1000.000000000000000 ) ;
#3966=FACE_OUTER_BOUND ( 'NONE', #5129, .T. ) ;
#3968=DIRECTION ( 'NONE',  ( 1.000000000000000000, 0.000000000000000000, 0.000000000000000000 ) ) ;
#3969=VECTOR ( 'NONE', #3888, 1000.000000000000000 ) ;
#3972=AXIS2_PLACEMENT_3D ( 'NONE', #2474, #1204, #3061 ) ;
#3981=AXIS2_PLACEMENT_3D ( 'NONE', #5900, #5940, #5420 ) ;
#3982=VECTOR ( 'NONE', #3679, 1000.000000000000000 ) ;
#3983=DIRECTION ( 'NONE',  ( 0.000000000000000000, 0.000000000000000000, -1.000000000000000000 ) ) ;
#3990=DIRECTION ( 'NONE',  ( 0.000000000000000000, 0.000000000000000000, -1.000000000000000000 ) ) ;
#3995=VECTOR ( 'NONE', #4549, 1000.000000000000000 ) ;
#3997=AXIS2_PLACEMENT_3D ( 'NONE', #90, #66, #124 ) ;
#3998=EDGE_CURVE ( 'NONE', #5323, #5207, #4085, .T. ) ;
#4006=CARTESIAN_POINT ( 'NONE',  ( 25.00000000000000711, -6.999999999999988454, -65.00000000000000000 ) ) ;
#4018=DIRECTION ( 'NONE',  ( 1.000000000000000000, -3.469446951953614189E-16, 0.000000000000000000 ) ) ;
#4022=ADVANCED_FACE ( 'NONE', ( #3149 ), #833, .F. ) ;
#4030=EDGE_CURVE ( 'NONE', #4855, #2228, #2372, .T. ) ;
#4038=ORIENTED_EDGE ( 'NONE', *, *, #4509, .F. ) ;
#4041=ORIENTED_EDGE ( 'NONE', *, *, #5570, .F. ) ;
#4046=ORIENTED_EDGE ( 'NONE', *, *, #4511, .T. ) ;
#4053=CARTESIAN_POINT ( 'NONE',  ( -45.00000000000001421, 15.00000000000000000, 45.00000000000000000 ) ) ;
#4060=ORIENTED_EDGE ( 'NONE', *, *, #876, .T. ) ;
#4065=EDGE_CURVE ( 'NONE', #782, #1576, #5063, .T. ) ;
#4067=AXIS2_PLACEMENT_3D ( 'NONE', #5265, #1555, #2984 ) ;
#4068=VECTOR ( 'NONE', #2281, 1000.000000000000000 ) ;
#4075=ORIENTED_EDGE ( 'NONE', *, *, #4507, .T. ) ;
#4076=PLANE ( 'NONE',  #2919 ) ;
#4084=AXIS2_PLACEMENT_3D ( 'NONE', #1501, #238, #5303 ) ;
#4085=CIRCLE ( 'NONE', #5351, 2.500000000000002220 ) ;
#4087=DIRECTION ( 'NONE',  ( 1.000000000000000000, -0.000000000000000000, -0.000000000000000000 ) ) ;
#4090=EDGE_LOOP ( 'NONE', ( #1186, #3375, #1581, #3193 ) ) ;
#4092=AXIS2_PLACEMENT_3D ( 'NONE', #4620, #3700, #5575 ) ;
#4097=ADVANCED_FACE ( 'NONE', ( #3263 ), #1280, .F. ) ;
#4100=FACE_BOUND ( 'NONE', #3360, .T. ) ;
#4102=LINE ( 'NONE', #1848, #5359 ) ;
#4103=CARTESIAN_POINT ( 'NONE',  ( -45.00000000000001421, 0.000000000000000000, 39.99999999999999289 ) ) ;
#4105=ORIENTED_EDGE ( 'NONE', *, *, #1022, .T. ) ;
#4106=EDGE_CURVE ( 'NONE', #283, #5207, #2710, .T. ) ;
#4107=ORIENTED_EDGE ( 'NONE', *, *, #5316, .F. ) ;
#4108=VECTOR ( 'NONE', #3279, 1000.000000000000000 ) ;
#4113=VECTOR ( 'NONE', #5165, 1000.000000000000000 ) ;
#4117=CARTESIAN_POINT ( 'NONE',  ( -74.99999999999998579, 15.00000000000000000, 75.00000000000000000 ) ) ;
#4127=AXIS2_PLACEMENT_3D ( 'NONE', #3576, #398, #2240 ) ;
#4128=CYLINDRICAL_SURFACE ( 'NONE', #4914, 7.000000000000000000 ) ;
#4129=ORIENTED_EDGE ( 'NONE', *, *, #3104, .T. ) ;
#4136=ORIENTED_EDGE ( 'NONE', *, *, #2899, .T. ) ;
#4149=CARTESIAN_POINT ( 'NONE',  ( 67.00000000000000000, 0.000000000000000000, -10.49999999999999822 ) ) ;
#4152=PLANE ( 'NONE',  #4279 ) ;
#4158=CARTESIAN_POINT ( 'NONE',  ( -45.00000000000002842, 15.00000000000000000, -49.99999999999998579 ) ) ;
#4173=DIRECTION ( 'NONE',  ( -0.000000000000000000, -0.000000000000000000, 1.000000000000000000 ) ) ;
#4176=CIRCLE ( 'NONE', #3685, 2.500000000000002220 ) ;
#4180=CONICAL_SURFACE ( 'NONE', #5238, 2.500000000000002220, 1.029744260000002631 ) ;
#4181=LINE ( 'NONE', #2866, #4667 ) ;
#4183=FACE_OUTER_BOUND ( 'NONE', #891, .T. ) ;
#4197=COLOUR_RGB ( '',0.8941176470588234615, 0.8941176470588234615, 0.8941176470588234615 ) ;
#4199=FACE_OUTER_BOUND ( 'NONE', #3858, .T. ) ;
#4203=DIRECTION ( 'NONE',  ( -1.000000000000000000, 0.000000000000000000, 0.000000000000000000 ) ) ;
#4209=VERTEX_POINT ( 'NONE', #1032 ) ;
#4216=CARTESIAN_POINT ( 'NONE',  ( 25.00000000000000711, 1.734723475976807094E-14, 0.000000000000000000 ) ) ;
#4227=VERTEX_POINT ( 'NONE', #3760 ) ;
#4229=DIRECTION ( 'NONE',  ( -0.000000000000000000, -1.000000000000000000, -0.000000000000000000 ) ) ;
#4246=DIRECTION ( 'NONE',  ( -0.000000000000000000, -0.000000000000000000, -1.000000000000000000 ) ) ;
#4251=ORIENTED_EDGE ( 'NONE', *, *, #2050, .T. ) ;
#4252=ORIENTED_EDGE ( 'NONE', *, *, #2086, .F. ) ;
#4254=MANIFOLD_SOLID_BREP ( 'AdvancedHole4', #3534 ) ;
#4256=DIRECTION ( 'NONE',  ( 0.000000000000000000, 0.000000000000000000, -1.000000000000000000 ) ) ;
#4260=DIRECTION ( 'NONE',  ( -0.000000000000000000, -0.000000000000000000, -1.000000000000000000 ) ) ;
#4261=AXIS2_PLACEMENT_3D ( 'NONE', #3741, #28, #3719 ) ;
#4264=ORIENTED_EDGE ( 'NONE', *, *, #5498, .F. ) ;
#4269=CARTESIAN_POINT ( 'NONE',  ( 25.00000000000000711, -6.999999999999989342, -75.00000000000000000 ) ) ;
#4272=EDGE_LOOP ( 'NONE', ( #5894, #2464 ) ) ;
#4279=AXIS2_PLACEMENT_3D ( 'NONE', #4727, #5075, #4638 ) ;
#4281=EDGE_LOOP ( 'NONE', ( #5398, #1648, #905, #5959 ) ) ;
#4283=UNCERTAINTY_MEASURE_WITH_UNIT (LENGTH_MEASURE( 1.000000000000000082E-05 ), #1212, 'distance_accuracy_value', 'NONE');
#4284=AXIS2_PLACEMENT_3D ( 'NONE', #2989, #3926, #2562 ) ;
#4286=ORIENTED_EDGE ( 'NONE', *, *, #2307, .F. ) ;
#4297=DIRECTION ( 'NONE',  ( -1.000000000000000000, 0.000000000000000000, 0.000000000000000000 ) ) ;
#4300=ORIENTED_EDGE ( 'NONE', *, *, #727, .T. ) ;
#4305=ORIENTED_EDGE ( 'NONE', *, *, #3277, .T. ) ;
#4315=EDGE_LOOP ( 'NONE', ( #273, #4952 ) ) ;
#4327=DIRECTION ( 'NONE',  ( -0.000000000000000000, -1.000000000000000000, -0.000000000000000000 ) ) ;
#4328=AXIS2_PLACEMENT_3D ( 'NONE', #1785, #847, #4987 ) ;
#4329=CARTESIAN_POINT ( 'NONE',  ( 25.00000000000000711, 7.000000000000011546, 75.00000000000000000 ) ) ;
#4336=ADVANCED_FACE ( 'NONE', ( #3194 ), #2698, .T. ) ;
#4339=CARTESIAN_POINT ( 'NONE',  ( 40.00000000000000711, 6.288372600415927295E-15, 55.00000000000000000 ) ) ;
#4340=CYLINDRICAL_SURFACE ( 'NONE', #3298, 2.500000000000002220 ) ;
#4342=ORIENTED_EDGE ( 'NONE', *, *, #1344, .T. ) ;
#4354=VERTEX_POINT ( 'NONE', #1814 ) ;
#4355=ADVANCED_FACE ( 'NONE', ( #4100, #402, #2732, #5081 ), #5883, .F. ) ;
#4364=CARTESIAN_POINT ( 'NONE',  ( 65.00000000000001421, -1.951563910473909559E-15, 65.00000000000000000 ) ) ;
#4367=DIRECTION ( 'NONE',  ( -0.000000000000000000, -0.000000000000000000, -1.000000000000000000 ) ) ;
#4374=LINE ( 'NONE', #3066, #3144 ) ;
#4375=EDGE_LOOP ( 'NONE', ( #3843, #183 ) ) ;
#4378=FILL_AREA_STYLE_COLOUR ( '', #4197 ) ;
#4379=CARTESIAN_POINT ( 'NONE',  ( 25.00000000000000711, 1.734723475976807094E-14, 0.000000000000000000 ) ) ;
#4387=CARTESIAN_POINT ( 'NONE',  ( 40.00000000000000711, 6.288372600415927295E-15, 65.00000000000000000 ) ) ;
#4393=CARTESIAN_POINT ( 'NONE',  ( 65.00000000000001421, -1.645402210687070900E-15, -55.00000000000000000 ) ) ;
#4394=ORIENTED_EDGE ( 'NONE', *, *, #1872, .T. ) ;
#4401=DIRECTION ( 'NONE',  ( -0.000000000000000000, -0.000000000000000000, -1.000000000000000000 ) ) ;
#4407=ORIENTED_EDGE ( 'NONE', *, *, #3387, .T. ) ;
#4409=DIRECTION ( 'NONE',  ( 0.000000000000000000, 1.000000000000000000, 0.000000000000000000 ) ) ;
#4413=CARTESIAN_POINT ( 'NONE',  ( 25.00000000000000711, 7.000000000000011546, 65.00000000000000000 ) ) ;
#4416=VERTEX_POINT ( 'NONE', #1846 ) ;
#4417=EDGE_LOOP ( 'NONE', ( #453, #898 ) ) ;
#4437=CYLINDRICAL_SURFACE ( 'NONE', #518, 2.500000000000002220 ) ;
#4438=EDGE_CURVE ( 'NONE', #2390, #5222, #125, .T. ) ;
#4441=PRESENTATION_STYLE_ASSIGNMENT (( #639 ) ) ;
#4443=DIRECTION ( 'NONE',  ( 0.000000000000000000, -1.000000000000000000, 0.000000000000000000 ) ) ;
#4444=VERTEX_POINT ( 'NONE', #4706 ) ;
#4447=DIRECTION ( 'NONE',  ( 0.000000000000000000, -1.000000000000000000, 0.000000000000000000 ) ) ;
#4450=CARTESIAN_POINT ( 'NONE',  ( 75.00000000000001421, 0.000000000000000000, -9.500000000000000000 ) ) ;
#4452=CARTESIAN_POINT ( 'NONE',  ( 75.00000000000001421, -7.000000000000006217, 65.00000000000000000 ) ) ;
#4463=CARTESIAN_POINT ( 'NONE',  ( 62.50000000000001421, -1.951563910473909559E-15, 65.00000000000000000 ) ) ;
#4468=VECTOR ( 'NONE', #1817, 1000.000000000000000 ) ;
#4472=EDGE_CURVE ( 'NONE', #2678, #1861, #5256, .T. ) ;
#4473=DIRECTION ( 'NONE',  ( 0.000000000000000000, 1.000000000000000000, 0.000000000000000000 ) ) ;
#4477=AXIS2_PLACEMENT_3D ( 'NONE', #3868, #2498, #1167 ) ;
#4485=VERTEX_POINT ( 'NONE', #1023 ) ;
#4487=ORIENTED_EDGE ( 'NONE', *, *, #3104, .F. ) ;
#4496=( GEOMETRIC_REPRESENTATION_CONTEXT ( 3 ) GLOBAL_UNCERTAINTY_ASSIGNED_CONTEXT ( ( #1540 ) ) GLOBAL_UNIT_ASSIGNED_CONTEXT ( ( #2550, #5767, #5348 ) ) REPRESENTATION_CONTEXT ( 'NONE', 'WORKASPACE' ) );
#4507=EDGE_CURVE ( 'NONE', #1345, #2273, #5104, .T. ) ;
#4509=EDGE_CURVE ( 'NONE', #5838, #3927, #5212, .T. ) ;
#4511=EDGE_CURVE ( 'NONE', #5507, #5437, #2301, .T. ) ;
#4525=ORIENTED_EDGE ( 'NONE', *, *, #1348, .F. ) ;
#4526=ADVANCED_FACE ( 'NONE', ( #1873 ), #3610, .F. ) ;
#4534=CARTESIAN_POINT ( 'NONE',  ( 67.00000000000000000, 1.224646799147353207E-16, 10.49999999999999822 ) ) ;
#4538=ORIENTED_EDGE ( 'NONE', *, *, #5835, .T. ) ;
#4540=DIRECTION ( 'NONE',  ( 0.000000000000000000, 0.000000000000000000, -1.000000000000000000 ) ) ;
#4545=CARTESIAN_POINT ( 'NONE',  ( 37.50000000000000711, 6.288372600415927295E-15, 55.00000000000000000 ) ) ;
#4549=DIRECTION ( 'NONE',  ( 1.000000000000000000, -2.312964634635742895E-17, 0.000000000000000000 ) ) ;
#4557=VECTOR ( 'NONE', #5465, 1000.000000000000000 ) ;
#4558=CARTESIAN_POINT ( 'NONE',  ( -45.00000000000001421, 0.000000000000000000, 45.00000000000000000 ) ) ;
#4567=DIRECTION ( 'NONE',  ( 1.000000000000000000, 0.000000000000000000, 0.000000000000000000 ) ) ;
#4568=EDGE_LOOP ( 'NONE', ( #3074, #1211 ) ) ;
#4574=AXIS2_PLACEMENT_3D ( 'NONE', #5890, #4936, #1737 ) ;
#4583=ORIENTED_EDGE ( 'NONE', *, *, #971, .F. ) ;
#4586=EDGE_CURVE ( 'NONE', #1041, #5450, #3873, .T. ) ;
#4594=DIRECTION ( 'NONE',  ( 0.000000000000000000, 0.000000000000000000, 1.000000000000000000 ) ) ;
#4609=CARTESIAN_POINT ( 'NONE',  ( 65.00000000000001421, -1.645402210687070900E-15, -55.00000000000000000 ) ) ;
#4618=DIRECTION ( 'NONE',  ( 1.000000000000000000, -0.000000000000000000, -0.000000000000000000 ) ) ;
#4620=CARTESIAN_POINT ( 'NONE',  ( 62.50000000000001421, -1.951563910473909559E-15, -55.00000000000000000 ) ) ;
#4632=ORIENTED_EDGE ( 'NONE', *, *, #2307, .T. ) ;
#4638=DIRECTION ( 'NONE',  ( -1.000000000000000000, 3.469446951953614189E-16, 0.000000000000000000 ) ) ;
#4639=ORIENTED_EDGE ( 'NONE', *, *, #640, .F. ) ;
#4642=DIRECTION ( 'NONE',  ( 1.000000000000000000, -2.312964634635742895E-17, 0.000000000000000000 ) ) ;
#4643=EDGE_LOOP ( 'NONE', ( #1463, #166, #3947, #326 ) ) ;
#4645=CARTESIAN_POINT ( 'NONE',  ( 65.00000000000001421, -1.951563910473909559E-15, 55.00000000000000000 ) ) ;
#4646=AXIS2_PLACEMENT_3D ( 'NONE', #2006, #2929, #2892 ) ;
#4652=CARTESIAN_POINT ( 'NONE',  ( 75.00000000000001421, 6.999999999999993783, -65.00000000000000000 ) ) ;
#4653=EDGE_CURVE ( 'NONE', #2273, #4783, #1111, .T. ) ;
#4664=EDGE_CURVE ( 'NONE', #5207, #5323, #688, .T. ) ;
#4666=AXIS2_PLACEMENT_3D ( 'NONE', #4216, #2407, #59 ) ;
#4667=VECTOR ( 'NONE', #558, 1000.000000000000114 ) ;
#4670=CARTESIAN_POINT ( 'NONE',  ( 65.00000000000001421, -1.645402210687070900E-15, -65.00000000000000000 ) ) ;
#4694=EDGE_CURVE ( 'NONE', #5475, #3671, #4760, .T. ) ;
#4698=LINE ( 'NONE', #1834, #5701 ) ;
#4706=CARTESIAN_POINT ( 'NONE',  ( -45.00000000000002842, 0.000000000000000000, -39.99999999999997868 ) ) ;
#4707=ADVANCED_FACE ( 'NONE', ( #632 ), #215, .F. ) ;
#4715=DIRECTION ( 'NONE',  ( 0.5150380737757185301, 1.049727191973310571E-16, 0.8571673013836900168 ) ) ;
#4717=CARTESIAN_POINT ( 'NONE',  ( 75.00000000000001421, -15.00000000000000355, 75.00000000000000000 ) ) ;
#4727=CARTESIAN_POINT ( 'NONE',  ( 25.00000000000000711, 7.000000000000011546, -65.00000000000000000 ) ) ;
#4741=CARTESIAN_POINT ( 'NONE',  ( 62.50000000000001421, -1.951563910473909559E-15, 55.00000000000000000 ) ) ;
#4749=ORIENTED_EDGE ( 'NONE', *, *, #4030, .F. ) ;
#4760=LINE ( 'NONE', #3841, #5914 ) ;
#4761=ADVANCED_FACE ( 'NONE', ( #815 ), #1749, .F. ) ;
#4763=VECTOR ( 'NONE', #2297, 1000.000000000000000 ) ;
#4765=EDGE_CURVE ( 'NONE', #1699, #3406, #1752, .T. ) ;
#4772=ORIENTED_EDGE ( 'NONE', *, *, #55, .F. ) ;
#4775=DIRECTION ( 'NONE',  ( -0.000000000000000000, -0.000000000000000000, 1.000000000000000000 ) ) ;
#4782=CYLINDRICAL_SURFACE ( 'NONE', #5704, 2.500000000000002220 ) ;
#4783=VERTEX_POINT ( 'NONE', #5488 ) ;
#4784=PLANE ( 'NONE',  #1452 ) ;
#4785=CARTESIAN_POINT ( 'NONE',  ( 25.00000000000000711, 7.000000000000011546, -65.00000000000000000 ) ) ;
#4788=ORIENTED_EDGE ( 'NONE', *, *, #2604, .T. ) ;
#4793=CARTESIAN_POINT ( 'NONE',  ( 25.00000000000000711, -6.999999999999988454, 65.00000000000000000 ) ) ;
#4802=( LENGTH_UNIT ( ) NAMED_UNIT ( * ) SI_UNIT ( .MILLI., .METRE. ) );
#4804=CARTESIAN_POINT ( 'NONE',  ( 67.00000000000000000, 1.224646799147353207E-16, -8.500000000000000000 ) ) ;
#4817=ORIENTED_EDGE ( 'NONE', *, *, #2764, .F. ) ;
#4821=CARTESIAN_POINT ( 'NONE',  ( 25.00000000000000711, -6.999999999999989342, 75.00000000000000000 ) ) ;
#4823=CARTESIAN_POINT ( 'NONE',  ( 75.00000000000001421, -15.00000000000000355, 75.00000000000000000 ) ) ;
#4830=ORIENTED_EDGE ( 'NONE', *, *, #1389, .T. ) ;
#4831=DIRECTION ( 'NONE',  ( 0.000000000000000000, 0.000000000000000000, 1.000000000000000000 ) ) ;
#4832=DIRECTION ( 'NONE',  ( 1.000000000000000000, -3.469446951953614189E-16, -0.000000000000000000 ) ) ;
#4835=ORIENTED_EDGE ( 'NONE', *, *, #3788, .F. ) ;
#4838=DIRECTION ( 'NONE',  ( 1.000000000000000000, -0.000000000000000000, -0.000000000000000000 ) ) ;
#4841=DIRECTION ( 'NONE',  ( -1.000000000000000000, 0.000000000000000000, -0.000000000000000000 ) ) ;
#4846=ADVANCED_FACE ( 'NONE', ( #3572 ), #5875, .F. ) ;
#4854=CARTESIAN_POINT ( 'NONE',  ( 62.50000000000001421, -1.951563910473909559E-15, -55.00000000000000000 ) ) ;
#4855=VERTEX_POINT ( 'NONE', #750 ) ;
#4856=EDGE_CURVE ( 'NONE', #1175, #736, #2518, .T. ) ;
#4860=CIRCLE ( 'NONE', #3697, 0.9999999999999991118 ) ;
#4866=VECTOR ( 'NONE', #1343, 1000.000000000000000 ) ;
#4873=AXIS2_PLACEMENT_3D ( 'NONE', #436, #4401, #2737 ) ;
#4874=AXIS2_PLACEMENT_3D ( 'NONE', #1029, #3282, #2396 ) ;
#4877=EDGE_CURVE ( 'NONE', #4354, #5437, #1917, .T. ) ;
#4879=DIRECTION ( 'NONE',  ( -0.000000000000000000, -0.000000000000000000, 1.000000000000000000 ) ) ;
#4884=ORIENTED_EDGE ( 'NONE', *, *, #2088, .T. ) ;
#4893=CARTESIAN_POINT ( 'NONE',  ( 25.00000000000000711, -6.999999999999988454, 65.00000000000000000 ) ) ;
#4899=ORIENTED_EDGE ( 'NONE', *, *, #5604, .T. ) ;
#4906=DIRECTION ( 'NONE',  ( -0.000000000000000000, -0.000000000000000000, -1.000000000000000000 ) ) ;
#4914=AXIS2_PLACEMENT_3D ( 'NONE', #5904, #4618, #5017 ) ;
#4918=DIRECTION ( 'NONE',  ( -0.000000000000000000, -1.000000000000000000, -0.000000000000000000 ) ) ;
#4920=CARTESIAN_POINT ( 'NONE',  ( 40.00000000000000711, 6.594534300202765954E-15, -55.00000000000000000 ) ) ;
#4921=DIRECTION ( 'NONE',  ( -0.000000000000000000, -0.000000000000000000, 1.000000000000000000 ) ) ;
#4924=FACE_OUTER_BOUND ( 'NONE', #2151, .T. ) ;
#4925=ORIENTED_EDGE ( 'NONE', *, *, #5234, .F. ) ;
#4936=DIRECTION ( 'NONE',  ( 1.000000000000000000, 0.000000000000000000, 0.000000000000000000 ) ) ;
#4951=AXIS2_PLACEMENT_3D ( 'NONE', #5958, #4203, #2798 ) ;
#4952=ORIENTED_EDGE ( 'NONE', *, *, #1344, .F. ) ;
#4955=ADVANCED_FACE ( 'NONE', ( #4183 ), #4152, .F. ) ;
#4961=DIRECTION ( 'NONE',  ( -1.000000000000000000, 0.000000000000000000, 0.000000000000000000 ) ) ;
#4965=AXIS2_PLACEMENT_3D ( 'NONE', #2967, #245, #1203 ) ;
#4972=EDGE_CURVE ( 'NONE', #5207, #3560, #5544, .T. ) ;
#4987=DIRECTION ( 'NONE',  ( 0.000000000000000000, -0.000000000000000000, -1.000000000000000000 ) ) ;
#4995=EDGE_CURVE ( 'NONE', #554, #726, #3, .T. ) ;
#4996=LINE ( 'NONE', #3557, #2811 ) ;
#4997=ADVANCED_FACE ( 'NONE', ( #507 ), #2356, .T. ) ;
#4999=VERTEX_POINT ( 'NONE', #5180 ) ;
#5000=DIRECTION ( 'NONE',  ( -1.000000000000000000, 0.000000000000000000, -0.000000000000000000 ) ) ;
#5001=AXIS2_PLACEMENT_3D ( 'NONE', #3709, #1398, #5000 ) ;
#5015=EDGE_LOOP ( 'NONE', ( #3455, #4129, #3563 ) ) ;
#5017=DIRECTION ( 'NONE',  ( 0.000000000000000000, 0.000000000000000000, -1.000000000000000000 ) ) ;
#5022=CARTESIAN_POINT ( 'NONE',  ( 75.00000000000001421, 1.224646799147354440E-16, 10.49999999999999822 ) ) ;
#5025=ORIENTED_EDGE ( 'NONE', *, *, #2662, .T. ) ;
#5027=APPLICATION_CONTEXT ( 'automotive_design' ) ;
#5029=ORIENTED_EDGE ( 'NONE', *, *, #753, .F. ) ;
#5031=DIRECTION ( 'NONE',  ( -0.8571673013836870192, 0.000000000000000000, -0.5150380737757234151 ) ) ;
#5041=LINE ( 'NONE', #1719, #3776 ) ;
#5043=DIRECTION ( 'NONE',  ( 0.000000000000000000, 0.000000000000000000, -1.000000000000000000 ) ) ;
#5051=AXIS2_PLACEMENT_3D ( 'NONE', #2399, #4260, #3652 ) ;
#5060=DIRECTION ( 'NONE',  ( 1.000000000000000000, -0.000000000000000000, -0.000000000000000000 ) ) ;
#5061=ORIENTED_EDGE ( 'NONE', *, *, #1022, .F. ) ;
#5063=LINE ( 'NONE', #1859, #2245 ) ;
#5075=DIRECTION ( 'NONE',  ( 3.469446951953614189E-16, 1.000000000000000000, -1.734723475976808327E-16 ) ) ;
#5080=AXIS2_PLACEMENT_3D ( 'NONE', #3527, #4831, #667 ) ;
#5081=FACE_OUTER_BOUND ( 'NONE', #1960, .T. ) ;
#5089=CARTESIAN_POINT ( 'NONE',  ( 66.39913938277356920, 0.000000000000000000, 9.500000000000000000 ) ) ;
#5092=CARTESIAN_POINT ( 'NONE',  ( 65.00000000000001421, -1.645402210687070900E-15, -65.00000000000000000 ) ) ;
#5094=VERTEX_POINT ( 'NONE', #1626 ) ;
#5096=FACE_OUTER_BOUND ( 'NONE', #2428, .T. ) ;
#5098=DIRECTION ( 'NONE',  ( 0.000000000000000000, 1.000000000000000000, 0.000000000000000000 ) ) ;
#5101=ORIENTED_EDGE ( 'NONE', *, *, #4509, .T. ) ;
#5103=CARTESIAN_POINT ( 'NONE',  ( 37.50000000000000711, 6.288372600415927295E-15, -55.00000000000000000 ) ) ;
#5104=LINE ( 'NONE', #2787, #228 ) ;
#5111=DIRECTION ( 'NONE',  ( 1.000000000000000000, -0.000000000000000000, -0.000000000000000000 ) ) ;
#5113=DIRECTION ( 'NONE',  ( -1.000000000000000000, 0.000000000000000000, -0.000000000000000000 ) ) ;
#5115=DIRECTION ( 'NONE',  ( -0.000000000000000000, -0.000000000000000000, 1.000000000000000000 ) ) ;
#5125=ORIENTED_EDGE ( 'NONE', *, *, #4972, .T. ) ;
#5127=CARTESIAN_POINT ( 'NONE',  ( 75.00000000000001421, 0.000000000000000000, 0.000000000000000000 ) ) ;
#5128=DIRECTION ( 'NONE',  ( 0.000000000000000000, 0.000000000000000000, 1.000000000000000000 ) ) ;
#5129=EDGE_LOOP ( 'NONE', ( #2660, #428, #5965, #5029 ) ) ;
#5134=AXIS2_PLACEMENT_3D ( 'NONE', #5559, #5060, #1400 ) ;
#5137=EDGE_CURVE ( 'NONE', #4999, #3205, #1941, .T. ) ;
#5140=AXIS2_PLACEMENT_3D ( 'NONE', #4545, #1538, #5247 ) ;
#5142=VECTOR ( 'NONE', #734, 1000.000000000000114 ) ;
#5144=EDGE_LOOP ( 'NONE', ( #482, #1269, #2219, #3442 ) ) ;
#5146=ORIENTED_EDGE ( 'NONE', *, *, #3762, .F. ) ;
#5148=CONICAL_SURFACE ( 'NONE', #205, 2.500000000000002220, 1.029744260000002631 ) ;
#5150=EDGE_CURVE ( 'NONE', #5607, #4227, #1160, .T. ) ;
#5151=DIRECTION ( 'NONE',  ( 0.000000000000000000, 1.000000000000000000, 0.000000000000000000 ) ) ;
#5162=AXIS2_PLACEMENT_3D ( 'NONE', #4558, #1241, #788 ) ;
#5163=ORIENTED_EDGE ( 'NONE', *, *, #3862, .F. ) ;
#5165=DIRECTION ( 'NONE',  ( 1.000000000000000000, -3.469446951953614189E-16, 0.000000000000000000 ) ) ;
#5167=LINE ( 'NONE', #3314, #5637 ) ;
#5171=FACE_OUTER_BOUND ( 'NONE', #1047, .T. ) ;
#5175=ORIENTED_EDGE ( 'NONE', *, *, #4995, .F. ) ;
#5177=DIRECTION ( 'NONE',  ( 0.000000000000000000, 1.000000000000000000, -0.000000000000000000 ) ) ;
#5180=CARTESIAN_POINT ( 'NONE',  ( 55.00000000000000711, 0.000000000000000000, -7.000000000000000000 ) ) ;
#5181=ORIENTED_EDGE ( 'NONE', *, *, #2504, .T. ) ;
#5184=CARTESIAN_POINT ( 'NONE',  ( 35.00000000000000000, 6.594534300202765954E-15, 65.00000000000000000 ) ) ;
#5185=VECTOR ( 'NONE', #3486, 1000.000000000000000 ) ;
#5186=LINE ( 'NONE', #2388, #5425 ) ;
#5189=PRODUCT_DEFINITION_SHAPE ( 'NONE', 'NONE',  #5537 ) ;
#5192=DIRECTION ( 'NONE',  ( -0.000000000000000000, -0.000000000000000000, 1.000000000000000000 ) ) ;
#5199=FACE_OUTER_BOUND ( 'NONE', #2292, .T. ) ;
#5201=EDGE_CURVE ( 'NONE', #3189, #4444, #2635, .T. ) ;
#5204=ADVANCED_FACE ( 'NONE', ( #1982 ), #3402, .F. ) ;
#5207=VERTEX_POINT ( 'NONE', #4393 ) ;
#5208=ADVANCED_FACE ( 'NONE', ( #5687 ), #2078, .F. ) ;
#5211=CARTESIAN_POINT ( 'NONE',  ( 75.00000000000001421, -7.000000000000006217, -65.00000000000000000 ) ) ;
#5212=LINE ( 'NONE', #512, #2249 ) ;
#5214=ORIENTED_EDGE ( 'NONE', *, *, #727, .F. ) ;
#5222=VERTEX_POINT ( 'NONE', #2224 ) ;
#5228=FACE_BOUND ( 'NONE', #4568, .T. ) ;
#5232=VECTOR ( 'NONE', #4473, 1000.000000000000000 ) ;
#5234=EDGE_CURVE ( 'NONE', #4416, #5838, #2589, .T. ) ;
#5236=DIRECTION ( 'NONE',  ( 0.000000000000000000, 1.000000000000000000, 0.000000000000000000 ) ) ;
#5238=AXIS2_PLACEMENT_3D ( 'NONE', #2757, #1296, #1835 ) ;
#5242=EDGE_CURVE ( 'NONE', #3560, #5481, #25, .T. ) ;
#5247=DIRECTION ( 'NONE',  ( 1.000000000000000000, 0.000000000000000000, 0.000000000000000000 ) ) ;
#5251=UNCERTAINTY_MEASURE_WITH_UNIT (LENGTH_MEASURE( 1.000000000000000082E-05 ), #4802, 'distance_accuracy_value', 'NONE');
#5256=CIRCLE ( 'NONE', #2740, 5.000000000000004441 ) ;
#5265=CARTESIAN_POINT ( 'NONE',  ( 25.00000000000000711, -6.999999999999988454, 65.00000000000000000 ) ) ;
#5269=SHAPE_REPRESENTATION ( 'Reciprocating Feed Carriage Block', ( #5080 ), #2935 ) ;
#5270=CYLINDRICAL_SURFACE ( 'NONE', #2815, 0.9999999999999991118 ) ;
#5273=DIRECTION ( 'NONE',  ( -0.000000000000000000, -0.000000000000000000, -1.000000000000000000 ) ) ;
#5274=AXIS2_PLACEMENT_3D ( 'NONE', #4006, #306, #1141 ) ;
#5292=CARTESIAN_POINT ( 'NONE',  ( 25.00000000000000711, -6.999999999999989342, 75.00000000000000000 ) ) ;
#5301=EDGE_CURVE ( 'NONE', #2228, #3393, #1197, .T. ) ;
#5302=DIRECTION ( 'NONE',  ( -1.000000000000000000, 0.000000000000000000, 0.000000000000000000 ) ) ;
#5303=DIRECTION ( 'NONE',  ( 0.000000000000000000, 0.000000000000000000, -1.000000000000000000 ) ) ;
#5313=FACE_BOUND ( 'NONE', #856, .T. ) ;
#5316=EDGE_CURVE ( 'NONE', #2003, #3927, #383, .T. ) ;
#5317=DIRECTION ( 'NONE',  ( -0.000000000000000000, 8.673617379884040402E-17, -1.000000000000000000 ) ) ;
#5319=EDGE_CURVE ( 'NONE', #2440, #475, #5389, .T. ) ;
#5323=VERTEX_POINT ( 'NONE', #3082 ) ;
#5325=DIRECTION ( 'NONE',  ( -0.000000000000000000, -0.000000000000000000, 1.000000000000000000 ) ) ;
#5326=VERTEX_POINT ( 'NONE', #5480 ) ;
#5330=DIRECTION ( 'NONE',  ( 1.000000000000000000, 0.000000000000000000, 0.000000000000000000 ) ) ;
#5332=CIRCLE ( 'NONE', #5134, 0.9999999999999991118 ) ;
#5336=FACE_OUTER_BOUND ( 'NONE', #4643, .T. ) ;
#5337=AXIS2_PLACEMENT_3D ( 'NONE', #3960, #2568, #1664 ) ;
#5348=( NAMED_UNIT ( * ) SI_UNIT ( $, .STERADIAN. ) SOLID_ANGLE_UNIT ( ) );
#5351=AXIS2_PLACEMENT_3D ( 'NONE', #2587, #1775, #3053 ) ;
#5352=CARTESIAN_POINT ( 'NONE',  ( 25.00000000000000711, -6.999999999999988454, -65.00000000000000000 ) ) ;
#5354=VERTEX_POINT ( 'NONE', #861 ) ;
#5358=CARTESIAN_POINT ( 'NONE',  ( 62.50000000000001421, -1.951563910473909559E-15, -65.00000000000000000 ) ) ;
#5359=VECTOR ( 'NONE', #1277, 1000.000000000000000 ) ;
#5380=CARTESIAN_POINT ( 'NONE',  ( 67.00000000000000000, 0.000000000000000000, 8.500000000000000000 ) ) ;
#5385=ORIENTED_EDGE ( 'NONE', *, *, #3998, .T. ) ;
#5389=LINE ( 'NONE', #1225, #2822 ) ;
#5390=VERTEX_POINT ( 'NONE', #4117 ) ;
#5391=EDGE_CURVE ( 'NONE', #283, #5323, #5508, .T. ) ;
#5394=CARTESIAN_POINT ( 'NONE',  ( 35.00000000000000000, 6.594534300202765954E-15, 55.00000000000000000 ) ) ;
#5397=DIRECTION ( 'NONE',  ( 1.000000000000000000, 0.000000000000000000, 0.000000000000000000 ) ) ;
#5398=ORIENTED_EDGE ( 'NONE', *, *, #5319, .T. ) ;
#5402=VERTEX_POINT ( 'NONE', #3364 ) ;
#5411=CARTESIAN_POINT ( 'NONE',  ( -45.00000000000001421, 15.00000000000000000, 50.00000000000000000 ) ) ;
#5413=ORIENTED_EDGE ( 'NONE', *, *, #388, .F. ) ;
#5420=DIRECTION ( 'NONE',  ( -1.000000000000000000, 0.000000000000000000, 0.000000000000000000 ) ) ;
#5425=VECTOR ( 'NONE', #1534, 1000.000000000000000 ) ;
#5433=AXIS2_PLACEMENT_3D ( 'NONE', #1743, #3598, #5728 ) ;
#5434=CIRCLE ( 'NONE', #1364, 2.500000000000002220 ) ;
#5437=VERTEX_POINT ( 'NONE', #5211 ) ;
#5445=CIRCLE ( 'NONE', #5926, 0.9999999999999991118 ) ;
#5447=LINE ( 'NONE', #356, #5828 ) ;
#5450=VERTEX_POINT ( 'NONE', #4793 ) ;
#5460=FACE_OUTER_BOUND ( 'NONE', #5015, .T. ) ;
#5464=AXIS2_PLACEMENT_3D ( 'NONE', #3396, #2879, #1512 ) ;
#5465=DIRECTION ( 'NONE',  ( 0.8571673013836870192, 0.000000000000000000, 0.5150380737757234151 ) ) ;
#5472=CARTESIAN_POINT ( 'NONE',  ( 75.00000000000001421, -15.00000000000000355, -75.00000000000000000 ) ) ;
#5473=VECTOR ( 'NONE', #4409, 1000.000000000000000 ) ;
#5475=VERTEX_POINT ( 'NONE', #1136 ) ;
#5480=CARTESIAN_POINT ( 'NONE',  ( 75.00000000000001421, 15.00000000000000000, 75.00000000000000000 ) ) ;
#5481=VERTEX_POINT ( 'NONE', #3906 ) ;
#5482=CARTESIAN_POINT ( 'NONE',  ( 67.00000000000000000, 0.000000000000000000, -9.500000000000000000 ) ) ;
#5488=CARTESIAN_POINT ( 'NONE',  ( 75.00000000000001421, -15.00000000000000355, -75.00000000000000000 ) ) ;
#5498=EDGE_CURVE ( 'NONE', #1875, #2650, #1600, .T. ) ;
#5507=VERTEX_POINT ( 'NONE', #3480 ) ;
#5508=LINE ( 'NONE', #5964, #4866 ) ;
#5509=ORIENTED_EDGE ( 'NONE', *, *, #1503, .F. ) ;
#5510=DIRECTION ( 'NONE',  ( 0.000000000000000000, -1.000000000000000000, 0.000000000000000000 ) ) ;
#5518=FACE_OUTER_BOUND ( 'NONE', #72, .T. ) ;
#5531=CARTESIAN_POINT ( 'NONE',  ( -45.00000000000002842, 15.00000000000000000, -49.99999999999998579 ) ) ;
#5537=PRODUCT_DEFINITION ( 'UNKNOWN', '', #5848, #2091 ) ;
#5538=VECTOR ( 'NONE', #5273, 1000.000000000000000 ) ;
#5539=VECTOR ( 'NONE', #19, 1000.000000000000000 ) ;
#5540=CARTESIAN_POINT ( 'NONE',  ( -45.00000000000002842, 15.00000000000000000, -44.99999999999998579 ) ) ;
#5544=LINE ( 'NONE', #4670, #705 ) ;
#5559=CARTESIAN_POINT ( 'NONE',  ( 67.00000000000000000, 0.000000000000000000, 9.500000000000000000 ) ) ;
#5560=EDGE_LOOP ( 'NONE', ( #146, #5699, #77, #251 ) ) ;
#5562=ORIENTED_EDGE ( 'NONE', *, *, #3582, .T. ) ;
#5564=DIRECTION ( 'NONE',  ( 0.000000000000000000, 0.000000000000000000, -1.000000000000000000 ) ) ;
#5567=DIRECTION ( 'NONE',  ( 1.000000000000000000, -0.000000000000000000, -0.000000000000000000 ) ) ;
#5570=EDGE_CURVE ( 'NONE', #702, #4783, #1323, .T. ) ;
#5575=DIRECTION ( 'NONE',  ( -1.000000000000000000, 0.000000000000000000, 0.000000000000000000 ) ) ;
#5581=CARTESIAN_POINT ( 'NONE',  ( 67.00000000000000000, 0.000000000000000000, 8.500000000000000000 ) ) ;
#5599=EDGE_CURVE ( 'NONE', #3406, #1699, #5732, .T. ) ;
#5600=VECTOR ( 'NONE', #5317, 1000.000000000000000 ) ;
#5604=EDGE_CURVE ( 'NONE', #2523, #1576, #33, .T. ) ;
#5606=AXIS2_PLACEMENT_3D ( 'NONE', #4741, #4775, #1616 ) ;
#5607=VERTEX_POINT ( 'NONE', #4920 ) ;
#5626=ORIENTED_EDGE ( 'NONE', *, *, #2548, .F. ) ;
#5637=VECTOR ( 'NONE', #2884, 1000.000000000000000 ) ;
#5639=DIRECTION ( 'NONE',  ( -1.000000000000000000, 3.469446951953614189E-16, 0.000000000000000000 ) ) ;
#5645=LINE ( 'NONE', #4534, #1546 ) ;
#5671=CARTESIAN_POINT ( 'NONE',  ( 25.00000000000000711, 7.000000000000011546, 65.00000000000000000 ) ) ;
#5685=CARTESIAN_POINT ( 'NONE',  ( 35.00000000000000000, 6.288372600415927295E-15, -65.00000000000000000 ) ) ;
#5686=LINE ( 'NONE', #1527, #1754 ) ;
#5687=FACE_OUTER_BOUND ( 'NONE', #1818, .T. ) ;
#5698=CARTESIAN_POINT ( 'NONE',  ( 75.00000000000001421, 15.00000000000000000, 75.00000000000000000 ) ) ;
#5699=ORIENTED_EDGE ( 'NONE', *, *, #2535, .T. ) ;
#5701=VECTOR ( 'NONE', #1466, 1000.000000000000000 ) ;
#5702=LINE ( 'NONE', #1548, #2480 ) ;
#5704=AXIS2_PLACEMENT_3D ( 'NONE', #197, #5325, #1522 ) ;
#5707=PLANE ( 'NONE',  #4067 ) ;
#5708=LINE ( 'NONE', #1591, #386 ) ;
#5710=DIRECTION ( 'NONE',  ( 1.000000000000000000, -0.000000000000000000, -0.000000000000000000 ) ) ;
#5712=AXIS2_PLACEMENT_3D ( 'NONE', #2072, #4447, #3983 ) ;
#5728=DIRECTION ( 'NONE',  ( 0.000000000000000000, 0.000000000000000000, -1.000000000000000000 ) ) ;
#5731=EDGE_CURVE ( 'NONE', #554, #5930, #5445, .T. ) ;
#5732=CIRCLE ( 'NONE', #3125, 5.000000000000004441 ) ;
#5736=MECHANICAL_DESIGN_GEOMETRIC_PRESENTATION_REPRESENTATION('',(#984),#1575);
#5752=CARTESIAN_POINT ( 'NONE',  ( 40.00000000000000711, 6.594534300202765954E-15, -65.00000000000000000 ) ) ;
#5764=LINE ( 'NONE', #2090, #5185 ) ;
#5767=( NAMED_UNIT ( * ) PLANE_ANGLE_UNIT ( ) SI_UNIT ( $, .RADIAN. ) );
#5768=CARTESIAN_POINT ( 'NONE',  ( 67.00000000000000000, 1.224646799147354440E-16, 10.49999999999999822 ) ) ;
#5773=ORIENTED_EDGE ( 'NONE', *, *, #4694, .T. ) ;
#5788=DIRECTION ( 'NONE',  ( -0.000000000000000000, -0.000000000000000000, -1.000000000000000000 ) ) ;
#5793=VERTEX_POINT ( 'NONE', #30 ) ;
#5806=FACE_OUTER_BOUND ( 'NONE', #1377, .T. ) ;
#5820=CARTESIAN_POINT ( 'NONE',  ( 75.00000000000001421, -7.000000000000006217, -65.00000000000000000 ) ) ;
#5827=VECTOR ( 'NONE', #2134, 1000.000000000000000 ) ;
#5828=VECTOR ( 'NONE', #1194, 1000.000000000000000 ) ;
#5834=ORIENTED_EDGE ( 'NONE', *, *, #1082, .F. ) ;
#5835=EDGE_CURVE ( 'NONE', #5354, #1426, #1464, .T. ) ;
#5836=FACE_OUTER_BOUND ( 'NONE', #4090, .T. ) ;
#5838=VERTEX_POINT ( 'NONE', #903 ) ;
#5842=ORIENTED_EDGE ( 'NONE', *, *, #3902, .T. ) ;
#5844=ORIENTED_EDGE ( 'NONE', *, *, #4877, .F. ) ;
#5848=PRODUCT_DEFINITION_FORMATION_WITH_SPECIFIED_SOURCE ( 'ANY', '', #58, .NOT_KNOWN. ) ;
#5851=CARTESIAN_POINT ( 'NONE',  ( -45.00000000000002842, 15.00000000000000000, -44.99999999999998579 ) ) ;
#5854=PLANE ( 'NONE',  #5274 ) ;
#5858=LINE ( 'NONE', #5380, #5142 ) ;
#5859=ORIENTED_EDGE ( 'NONE', *, *, #1503, .T. ) ;
#5870=ADVANCED_FACE ( 'NONE', ( #4199 ), #520, .F. ) ;
#5875=CYLINDRICAL_SURFACE ( 'NONE', #1457, 2.500000000000002220 ) ;
#5883=PLANE ( 'NONE',  #5927 ) ;
#5890=CARTESIAN_POINT ( 'NONE',  ( -74.99999999999998579, -15.00000000000000000, 75.00000000000000000 ) ) ;
#5894=ORIENTED_EDGE ( 'NONE', *, *, #3582, .F. ) ;
#5897=CARTESIAN_POINT ( 'NONE',  ( -45.00000000000001421, 15.00000000000000000, 39.99999999999999289 ) ) ;
#5900=CARTESIAN_POINT ( 'NONE',  ( 62.50000000000001421, -1.951563910473909559E-15, -65.00000000000000000 ) ) ;
#5904=CARTESIAN_POINT ( 'NONE',  ( 55.00000000000000711, 0.000000000000000000, 0.000000000000000000 ) ) ;
#5907=ORIENTED_EDGE ( 'NONE', *, *, #1010, .F. ) ;
#5911=CIRCLE ( 'NONE', #3399, 2.500000000000002220 ) ;
#5912=EDGE_CURVE ( 'NONE', #1699, #2678, #5167, .T. ) ;
#5914=VECTOR ( 'NONE', #603, 1000.000000000000000 ) ;
#5919=AXIS2_PLACEMENT_3D ( 'NONE', #743, #3567, #3181 ) ;
#5926=AXIS2_PLACEMENT_3D ( 'NONE', #2296, #5567, #1836 ) ;
#5927=AXIS2_PLACEMENT_3D ( 'NONE', #2763, #2643, #4594 ) ;
#5928=FACE_OUTER_BOUND ( 'NONE', #735, .T. ) ;
#5930=VERTEX_POINT ( 'NONE', #5581 ) ;
#5931=CARTESIAN_POINT ( 'NONE',  ( 35.00000000000000000, 6.288372600415927295E-15, -65.00000000000000000 ) ) ;
#5938=CARTESIAN_POINT ( 'NONE',  ( -45.00000000000001421, 15.00000000000000000, 45.00000000000000000 ) ) ;
#5940=DIRECTION ( 'NONE',  ( -0.000000000000000000, -0.000000000000000000, -1.000000000000000000 ) ) ;
#5947=ADVANCED_FACE ( 'NONE', ( #1004 ), #1181, .F. ) ;
#5952=CARTESIAN_POINT ( 'NONE',  ( 25.00000000000000711, 7.000000000000011546, -65.00000000000000000 ) ) ;
#5955=ORIENTED_EDGE ( 'NONE', *, *, #316, .T. ) ;
#5956=EDGE_LOOP ( 'NONE', ( #4525, #1497, #253, #3285 ) ) ;
#5958=CARTESIAN_POINT ( 'NONE',  ( 55.00000000000000711, -15.00000000000000355, 75.00000000000000000 ) ) ;
#5959=ORIENTED_EDGE ( 'NONE', *, *, #910, .T. ) ;
#5960=FACE_OUTER_BOUND ( 'NONE', #22, .T. ) ;
#5961=ADVANCED_FACE ( 'NONE', ( #100 ), #1935, .F. ) ;
#5964=CARTESIAN_POINT ( 'NONE',  ( 60.00000000000001421, -1.951563910473909559E-15, -55.00000000000000000 ) ) ;
#5965=ORIENTED_EDGE ( 'NONE', *, *, #3706, .T. ) ;
#5967=CARTESIAN_POINT ( 'NONE',  ( 75.00000000000001421, 0.000000000000000000, 9.500000000000000000 ) ) ;
#5969=CARTESIAN_POINT ( 'NONE',  ( 37.50000000000000711, 6.288372600415927295E-15, 65.00000000000000000 ) ) ;
#5971=CARTESIAN_POINT ( 'NONE',  ( 75.00000000000001421, -15.00000000000000355, 75.00000000000000000 ) ) ;
#5993=COLOUR_RGB('Dark Blue',0.08,0.2,0.34);
#5994=FILL_AREA_STYLE_COLOUR('',#5993);
#5995=FILL_AREA_STYLE('',(#5994));
#5996=SURFACE_STYLE_FILL_AREA(#5995);
#5997=SURFACE_SIDE_STYLE('',(#5996));
#5998=SURFACE_STYLE_USAGE(.BOTH.,#5997);
#5999=PRESENTATION_STYLE_ASSIGNMENT((#5998));
ENDSEC;
END-ISO-10303-21;
